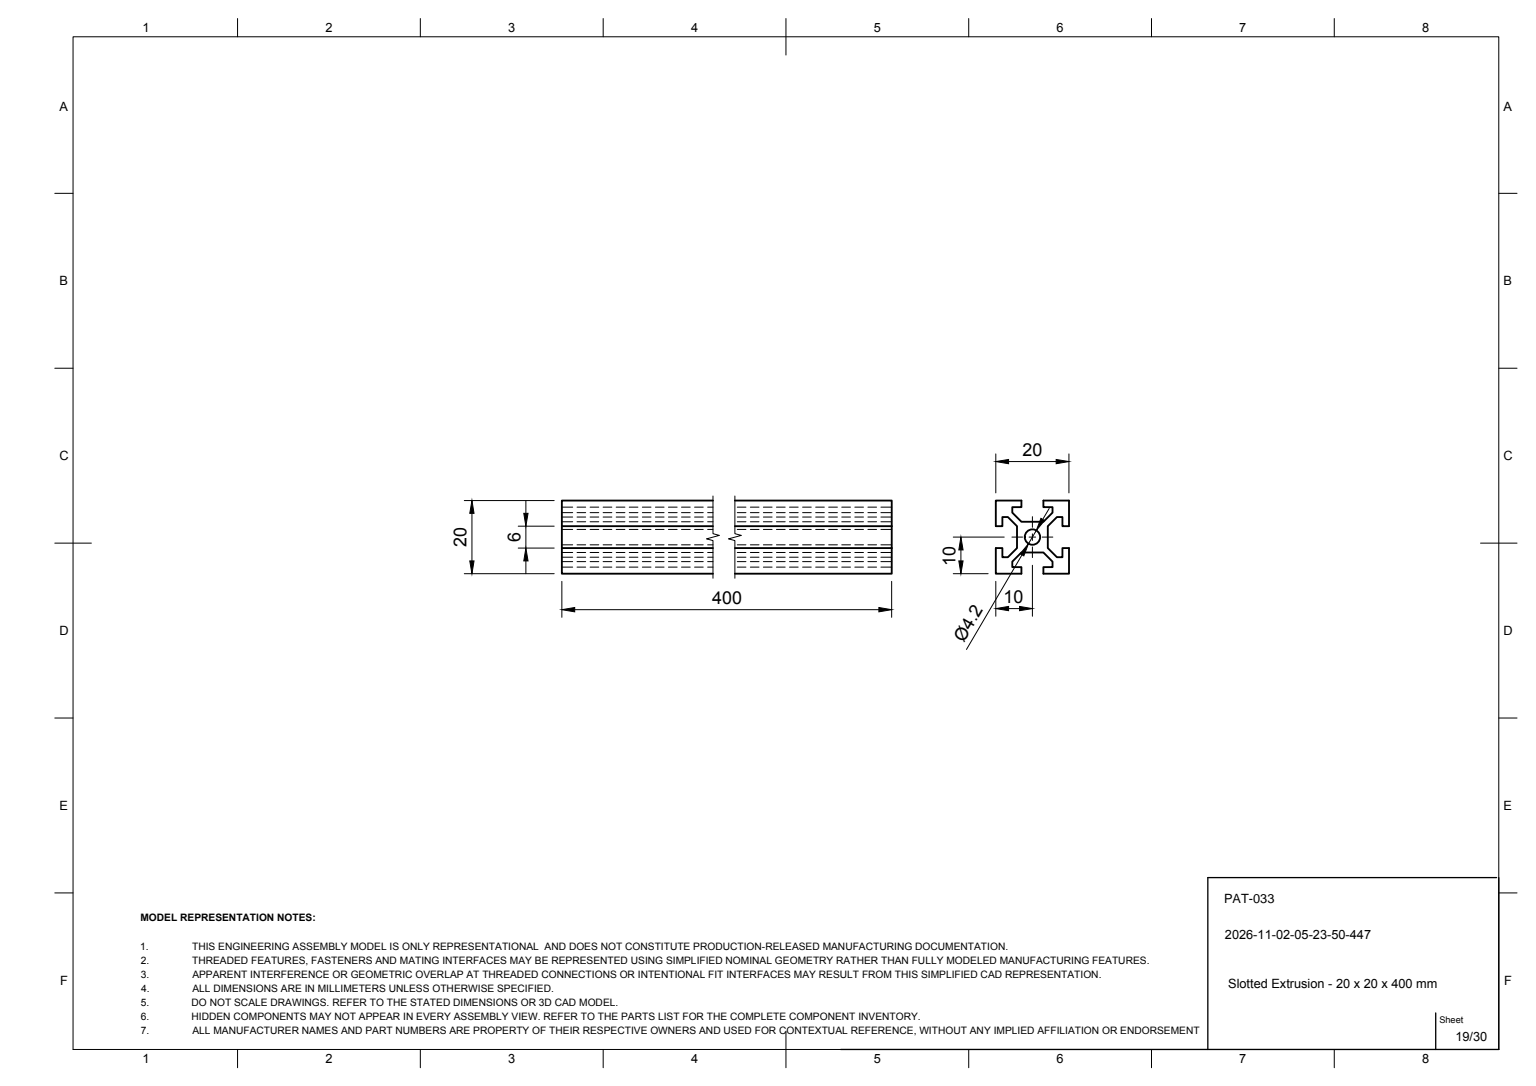
ISO-10303-21;
HEADER;
/* Generated by software containing ST-Developer
 * from STEP Tools, Inc. (www.steptools.com) 
 */

FILE_DESCRIPTION(
/* description */ ('Dual-rail gantry carriage'),
/* implementation_level */ '2;1');

FILE_NAME(
/* name */ 'Slotted Extrusion - 20 x 20 x 400 mm.step',
/* time_stamp */ '2026-10-27T10:49:15-07:00',
/* author */ (''),
/* organization */ (''),
/* preprocessor_version */ 'ST-DEVELOPER v20.2',
/* originating_system */ 'Autodesk Translation Framework v15.17.0.0',
/* authorisation */ '');

FILE_SCHEMA (('AUTOMOTIVE_DESIGN { 1 0 10303 214 3 1 1 }'));
ENDSEC;

DATA;
#10=MECHANICAL_DESIGN_GEOMETRIC_PRESENTATION_REPRESENTATION('',(#599),#12804);
#537=SHAPE_REPRESENTATION_RELATIONSHIP('SRR','None',#13015,#568);
#568=ADVANCED_BREP_SHAPE_REPRESENTATION('',(#630),#12785);
#599=STYLED_ITEM('',(#13233),#630);
#630=MANIFOLD_SOLID_BREP('Body1',#7377);
#690=FACE_BOUND('',#1655,.T.);
#691=FACE_BOUND('',#1657,.T.);
#856=PLANE('',#7946);
#857=PLANE('',#7947);
#858=PLANE('',#7948);
#859=PLANE('',#7949);
#860=PLANE('',#7950);
#861=PLANE('',#7951);
#862=PLANE('',#7952);
#863=PLANE('',#7953);
#864=PLANE('',#7954);
#865=PLANE('',#7955);
#866=PLANE('',#7956);
#867=PLANE('',#7957);
#868=PLANE('',#7958);
#869=PLANE('',#7959);
#870=PLANE('',#7960);
#871=PLANE('',#7961);
#872=PLANE('',#7962);
#873=PLANE('',#7963);
#874=PLANE('',#7964);
#875=PLANE('',#7965);
#876=PLANE('',#7966);
#877=PLANE('',#7967);
#878=PLANE('',#7968);
#879=PLANE('',#7969);
#880=PLANE('',#7970);
#881=PLANE('',#7971);
#882=PLANE('',#7972);
#883=PLANE('',#7973);
#884=PLANE('',#7974);
#885=PLANE('',#7975);
#886=PLANE('',#7976);
#887=PLANE('',#7977);
#888=PLANE('',#7978);
#889=PLANE('',#7979);
#890=PLANE('',#7980);
#891=PLANE('',#7981);
#892=PLANE('',#7985);
#893=PLANE('',#7986);
#894=PLANE('',#7987);
#895=PLANE('',#7988);
#896=PLANE('',#7989);
#897=PLANE('',#7990);
#898=PLANE('',#7991);
#899=PLANE('',#7992);
#900=PLANE('',#7993);
#901=PLANE('',#7994);
#1172=FACE_OUTER_BOUND('',#1609,.T.);
#1173=FACE_OUTER_BOUND('',#1610,.T.);
#1174=FACE_OUTER_BOUND('',#1611,.T.);
#1175=FACE_OUTER_BOUND('',#1612,.T.);
#1176=FACE_OUTER_BOUND('',#1613,.T.);
#1177=FACE_OUTER_BOUND('',#1614,.T.);
#1178=FACE_OUTER_BOUND('',#1615,.T.);
#1179=FACE_OUTER_BOUND('',#1616,.T.);
#1180=FACE_OUTER_BOUND('',#1617,.T.);
#1181=FACE_OUTER_BOUND('',#1618,.T.);
#1182=FACE_OUTER_BOUND('',#1619,.T.);
#1183=FACE_OUTER_BOUND('',#1620,.T.);
#1184=FACE_OUTER_BOUND('',#1621,.T.);
#1185=FACE_OUTER_BOUND('',#1622,.T.);
#1186=FACE_OUTER_BOUND('',#1623,.T.);
#1187=FACE_OUTER_BOUND('',#1624,.T.);
#1188=FACE_OUTER_BOUND('',#1625,.T.);
#1189=FACE_OUTER_BOUND('',#1626,.T.);
#1190=FACE_OUTER_BOUND('',#1627,.T.);
#1191=FACE_OUTER_BOUND('',#1628,.T.);
#1192=FACE_OUTER_BOUND('',#1629,.T.);
#1193=FACE_OUTER_BOUND('',#1630,.T.);
#1194=FACE_OUTER_BOUND('',#1631,.T.);
#1195=FACE_OUTER_BOUND('',#1632,.T.);
#1196=FACE_OUTER_BOUND('',#1633,.T.);
#1197=FACE_OUTER_BOUND('',#1634,.T.);
#1198=FACE_OUTER_BOUND('',#1635,.T.);
#1199=FACE_OUTER_BOUND('',#1636,.T.);
#1200=FACE_OUTER_BOUND('',#1637,.T.);
#1201=FACE_OUTER_BOUND('',#1638,.T.);
#1202=FACE_OUTER_BOUND('',#1639,.T.);
#1203=FACE_OUTER_BOUND('',#1640,.T.);
#1204=FACE_OUTER_BOUND('',#1641,.T.);
#1205=FACE_OUTER_BOUND('',#1642,.T.);
#1206=FACE_OUTER_BOUND('',#1643,.T.);
#1207=FACE_OUTER_BOUND('',#1644,.T.);
#1208=FACE_OUTER_BOUND('',#1645,.T.);
#1209=FACE_OUTER_BOUND('',#1646,.T.);
#1210=FACE_OUTER_BOUND('',#1647,.T.);
#1211=FACE_OUTER_BOUND('',#1648,.T.);
#1212=FACE_OUTER_BOUND('',#1649,.T.);
#1213=FACE_OUTER_BOUND('',#1650,.T.);
#1214=FACE_OUTER_BOUND('',#1651,.T.);
#1215=FACE_OUTER_BOUND('',#1652,.T.);
#1216=FACE_OUTER_BOUND('',#1653,.T.);
#1217=FACE_OUTER_BOUND('',#1654,.T.);
#1218=FACE_OUTER_BOUND('',#1656,.T.);
#1609=EDGE_LOOP('',(#5627,#5628,#5629,#5630));
#1610=EDGE_LOOP('',(#5631,#5632,#5633,#5634));
#1611=EDGE_LOOP('',(#5635,#5636,#5637,#5638));
#1612=EDGE_LOOP('',(#5639,#5640,#5641,#5642));
#1613=EDGE_LOOP('',(#5643,#5644,#5645,#5646));
#1614=EDGE_LOOP('',(#5647,#5648,#5649,#5650));
#1615=EDGE_LOOP('',(#5651,#5652,#5653,#5654));
#1616=EDGE_LOOP('',(#5655,#5656,#5657,#5658));
#1617=EDGE_LOOP('',(#5659,#5660,#5661,#5662));
#1618=EDGE_LOOP('',(#5663,#5664,#5665,#5666));
#1619=EDGE_LOOP('',(#5667,#5668,#5669,#5670));
#1620=EDGE_LOOP('',(#5671,#5672,#5673,#5674));
#1621=EDGE_LOOP('',(#5675,#5676,#5677,#5678));
#1622=EDGE_LOOP('',(#5679,#5680,#5681,#5682));
#1623=EDGE_LOOP('',(#5683,#5684,#5685,#5686));
#1624=EDGE_LOOP('',(#5687,#5688,#5689,#5690));
#1625=EDGE_LOOP('',(#5691,#5692,#5693,#5694));
#1626=EDGE_LOOP('',(#5695,#5696,#5697,#5698));
#1627=EDGE_LOOP('',(#5699,#5700,#5701,#5702));
#1628=EDGE_LOOP('',(#5703,#5704,#5705,#5706));
#1629=EDGE_LOOP('',(#5707,#5708,#5709,#5710));
#1630=EDGE_LOOP('',(#5711,#5712,#5713,#5714));
#1631=EDGE_LOOP('',(#5715,#5716,#5717,#5718));
#1632=EDGE_LOOP('',(#5719,#5720,#5721,#5722));
#1633=EDGE_LOOP('',(#5723,#5724,#5725,#5726));
#1634=EDGE_LOOP('',(#5727,#5728,#5729,#5730));
#1635=EDGE_LOOP('',(#5731,#5732,#5733,#5734));
#1636=EDGE_LOOP('',(#5735,#5736,#5737,#5738));
#1637=EDGE_LOOP('',(#5739,#5740,#5741,#5742));
#1638=EDGE_LOOP('',(#5743,#5744,#5745,#5746));
#1639=EDGE_LOOP('',(#5747,#5748,#5749,#5750));
#1640=EDGE_LOOP('',(#5751,#5752,#5753,#5754));
#1641=EDGE_LOOP('',(#5755,#5756,#5757,#5758));
#1642=EDGE_LOOP('',(#5759,#5760,#5761,#5762));
#1643=EDGE_LOOP('',(#5763,#5764,#5765,#5766));
#1644=EDGE_LOOP('',(#5767,#5768,#5769,#5770));
#1645=EDGE_LOOP('',(#5771,#5772,#5773,#5774));
#1646=EDGE_LOOP('',(#5775,#5776,#5777,#5778));
#1647=EDGE_LOOP('',(#5779,#5780,#5781,#5782));
#1648=EDGE_LOOP('',(#5783,#5784,#5785,#5786));
#1649=EDGE_LOOP('',(#5787,#5788,#5789,#5790));
#1650=EDGE_LOOP('',(#5791,#5792,#5793,#5794));
#1651=EDGE_LOOP('',(#5795,#5796,#5797,#5798));
#1652=EDGE_LOOP('',(#5799,#5800,#5801,#5802));
#1653=EDGE_LOOP('',(#5803,#5804,#5805,#5806));
#1654=EDGE_LOOP('',(#5807,#5808,#5809,#5810,#5811,#5812,#5813,#5814,#5815,
#5816,#5817,#5818,#5819,#5820,#5821,#5822,#5823,#5824,#5825,#5826,#5827,
#5828,#5829,#5830,#5831,#5832,#5833,#5834,#5835,#5836,#5837,#5838,#5839,
#5840,#5841,#5842,#5843,#5844,#5845,#5846,#5847,#5848,#5849,#5850));
#1655=EDGE_LOOP('',(#5851));
#1656=EDGE_LOOP('',(#5852,#5853,#5854,#5855,#5856,#5857,#5858,#5859,#5860,
#5861,#5862,#5863,#5864,#5865,#5866,#5867,#5868,#5869,#5870,#5871,#5872,
#5873,#5874,#5875,#5876,#5877,#5878,#5879,#5880,#5881,#5882,#5883,#5884,
#5885,#5886,#5887,#5888,#5889,#5890,#5891,#5892,#5893,#5894,#5895));
#1657=EDGE_LOOP('',(#5896));
#2164=LINE('',#11288,#2873);
#2165=LINE('',#11290,#2874);
#2166=LINE('',#11292,#2875);
#2167=LINE('',#11293,#2876);
#2168=LINE('',#11296,#2877);
#2169=LINE('',#11298,#2878);
#2170=LINE('',#11299,#2879);
#2171=LINE('',#11302,#2880);
#2172=LINE('',#11304,#2881);
#2173=LINE('',#11305,#2882);
#2174=LINE('',#11308,#2883);
#2175=LINE('',#11310,#2884);
#2176=LINE('',#11311,#2885);
#2177=LINE('',#11314,#2886);
#2178=LINE('',#11316,#2887);
#2179=LINE('',#11317,#2888);
#2180=LINE('',#11320,#2889);
#2181=LINE('',#11322,#2890);
#2182=LINE('',#11323,#2891);
#2183=LINE('',#11326,#2892);
#2184=LINE('',#11328,#2893);
#2185=LINE('',#11329,#2894);
#2186=LINE('',#11332,#2895);
#2187=LINE('',#11334,#2896);
#2188=LINE('',#11335,#2897);
#2189=LINE('',#11338,#2898);
#2190=LINE('',#11340,#2899);
#2191=LINE('',#11341,#2900);
#2192=LINE('',#11345,#2901);
#2193=LINE('',#11347,#2902);
#2194=LINE('',#11349,#2903);
#2195=LINE('',#11350,#2904);
#2196=LINE('',#11353,#2905);
#2197=LINE('',#11355,#2906);
#2198=LINE('',#11356,#2907);
#2199=LINE('',#11359,#2908);
#2200=LINE('',#11361,#2909);
#2201=LINE('',#11362,#2910);
#2202=LINE('',#11365,#2911);
#2203=LINE('',#11367,#2912);
#2204=LINE('',#11368,#2913);
#2205=LINE('',#11371,#2914);
#2206=LINE('',#11373,#2915);
#2207=LINE('',#11374,#2916);
#2208=LINE('',#11377,#2917);
#2209=LINE('',#11379,#2918);
#2210=LINE('',#11380,#2919);
#2211=LINE('',#11383,#2920);
#2212=LINE('',#11385,#2921);
#2213=LINE('',#11386,#2922);
#2214=LINE('',#11389,#2923);
#2215=LINE('',#11391,#2924);
#2216=LINE('',#11392,#2925);
#2217=LINE('',#11395,#2926);
#2218=LINE('',#11397,#2927);
#2219=LINE('',#11398,#2928);
#2220=LINE('',#11402,#2929);
#2221=LINE('',#11404,#2930);
#2222=LINE('',#11406,#2931);
#2223=LINE('',#11407,#2932);
#2224=LINE('',#11410,#2933);
#2225=LINE('',#11412,#2934);
#2226=LINE('',#11413,#2935);
#2227=LINE('',#11416,#2936);
#2228=LINE('',#11418,#2937);
#2229=LINE('',#11419,#2938);
#2230=LINE('',#11422,#2939);
#2231=LINE('',#11424,#2940);
#2232=LINE('',#11425,#2941);
#2233=LINE('',#11428,#2942);
#2234=LINE('',#11430,#2943);
#2235=LINE('',#11431,#2944);
#2236=LINE('',#11434,#2945);
#2237=LINE('',#11436,#2946);
#2238=LINE('',#11437,#2947);
#2239=LINE('',#11440,#2948);
#2240=LINE('',#11442,#2949);
#2241=LINE('',#11443,#2950);
#2242=LINE('',#11446,#2951);
#2243=LINE('',#11448,#2952);
#2244=LINE('',#11449,#2953);
#2245=LINE('',#11452,#2954);
#2246=LINE('',#11454,#2955);
#2247=LINE('',#11455,#2956);
#2248=LINE('',#11459,#2957);
#2249=LINE('',#11461,#2958);
#2250=LINE('',#11463,#2959);
#2251=LINE('',#11464,#2960);
#2252=LINE('',#11467,#2961);
#2253=LINE('',#11469,#2962);
#2254=LINE('',#11470,#2963);
#2255=LINE('',#11473,#2964);
#2256=LINE('',#11475,#2965);
#2257=LINE('',#11476,#2966);
#2258=LINE('',#11479,#2967);
#2259=LINE('',#11481,#2968);
#2260=LINE('',#11482,#2969);
#2261=LINE('',#11485,#2970);
#2262=LINE('',#11487,#2971);
#2263=LINE('',#11488,#2972);
#2264=LINE('',#11491,#2973);
#2265=LINE('',#11493,#2974);
#2266=LINE('',#11494,#2975);
#2267=LINE('',#11497,#2976);
#2268=LINE('',#11499,#2977);
#2269=LINE('',#11500,#2978);
#2270=LINE('',#11503,#2979);
#2271=LINE('',#11505,#2980);
#2272=LINE('',#11506,#2981);
#2273=LINE('',#11509,#2982);
#2274=LINE('',#11511,#2983);
#2275=LINE('',#11512,#2984);
#2276=LINE('',#11517,#2985);
#2277=LINE('',#11521,#2986);
#2278=LINE('',#11523,#2987);
#2279=LINE('',#11524,#2988);
#2280=LINE('',#11527,#2989);
#2281=LINE('',#11529,#2990);
#2282=LINE('',#11530,#2991);
#2283=LINE('',#11532,#2992);
#2284=LINE('',#11533,#2993);
#2285=LINE('',#11536,#2994);
#2286=LINE('',#11538,#2995);
#2287=LINE('',#11539,#2996);
#2288=LINE('',#11541,#2997);
#2289=LINE('',#11542,#2998);
#2290=LINE('',#11545,#2999);
#2291=LINE('',#11547,#3000);
#2292=LINE('',#11548,#3001);
#2293=LINE('',#11550,#3002);
#2294=LINE('',#11551,#3003);
#2295=LINE('',#11553,#3004);
#2296=LINE('',#11554,#3005);
#2873=VECTOR('',#9115,1.);
#2874=VECTOR('',#9116,1.);
#2875=VECTOR('',#9117,1.);
#2876=VECTOR('',#9118,1.);
#2877=VECTOR('',#9121,1.);
#2878=VECTOR('',#9122,1.);
#2879=VECTOR('',#9123,1.);
#2880=VECTOR('',#9126,1.);
#2881=VECTOR('',#9127,1.);
#2882=VECTOR('',#9128,1.);
#2883=VECTOR('',#9131,1.);
#2884=VECTOR('',#9132,1.);
#2885=VECTOR('',#9133,1.);
#2886=VECTOR('',#9136,1.);
#2887=VECTOR('',#9137,1.);
#2888=VECTOR('',#9138,1.);
#2889=VECTOR('',#9141,1.);
#2890=VECTOR('',#9142,1.);
#2891=VECTOR('',#9143,1.);
#2892=VECTOR('',#9146,1.);
#2893=VECTOR('',#9147,1.);
#2894=VECTOR('',#9148,1.);
#2895=VECTOR('',#9151,1.);
#2896=VECTOR('',#9152,1.);
#2897=VECTOR('',#9153,1.);
#2898=VECTOR('',#9156,1.);
#2899=VECTOR('',#9157,1.);
#2900=VECTOR('',#9158,1.);
#2901=VECTOR('',#9161,1.);
#2902=VECTOR('',#9162,1.);
#2903=VECTOR('',#9163,1.);
#2904=VECTOR('',#9164,1.);
#2905=VECTOR('',#9167,1.);
#2906=VECTOR('',#9168,1.);
#2907=VECTOR('',#9169,1.);
#2908=VECTOR('',#9172,1.);
#2909=VECTOR('',#9173,1.);
#2910=VECTOR('',#9174,1.);
#2911=VECTOR('',#9177,1.);
#2912=VECTOR('',#9178,1.);
#2913=VECTOR('',#9179,1.);
#2914=VECTOR('',#9182,1.);
#2915=VECTOR('',#9183,1.);
#2916=VECTOR('',#9184,1.);
#2917=VECTOR('',#9187,1.);
#2918=VECTOR('',#9188,1.);
#2919=VECTOR('',#9189,1.);
#2920=VECTOR('',#9192,1.);
#2921=VECTOR('',#9193,1.);
#2922=VECTOR('',#9194,1.);
#2923=VECTOR('',#9197,1.);
#2924=VECTOR('',#9198,1.);
#2925=VECTOR('',#9199,1.);
#2926=VECTOR('',#9202,1.);
#2927=VECTOR('',#9203,1.);
#2928=VECTOR('',#9204,1.);
#2929=VECTOR('',#9207,1.);
#2930=VECTOR('',#9208,1.);
#2931=VECTOR('',#9209,1.);
#2932=VECTOR('',#9210,1.);
#2933=VECTOR('',#9213,1.);
#2934=VECTOR('',#9214,1.);
#2935=VECTOR('',#9215,1.);
#2936=VECTOR('',#9218,1.);
#2937=VECTOR('',#9219,1.);
#2938=VECTOR('',#9220,1.);
#2939=VECTOR('',#9223,1.);
#2940=VECTOR('',#9224,1.);
#2941=VECTOR('',#9225,1.);
#2942=VECTOR('',#9228,1.);
#2943=VECTOR('',#9229,1.);
#2944=VECTOR('',#9230,1.);
#2945=VECTOR('',#9233,1.);
#2946=VECTOR('',#9234,1.);
#2947=VECTOR('',#9235,1.);
#2948=VECTOR('',#9238,1.);
#2949=VECTOR('',#9239,1.);
#2950=VECTOR('',#9240,1.);
#2951=VECTOR('',#9243,1.);
#2952=VECTOR('',#9244,1.);
#2953=VECTOR('',#9245,1.);
#2954=VECTOR('',#9248,1.);
#2955=VECTOR('',#9249,1.);
#2956=VECTOR('',#9250,1.);
#2957=VECTOR('',#9253,1.);
#2958=VECTOR('',#9254,1.);
#2959=VECTOR('',#9255,1.);
#2960=VECTOR('',#9256,1.);
#2961=VECTOR('',#9259,1.);
#2962=VECTOR('',#9260,1.);
#2963=VECTOR('',#9261,1.);
#2964=VECTOR('',#9264,1.);
#2965=VECTOR('',#9265,1.);
#2966=VECTOR('',#9266,1.);
#2967=VECTOR('',#9269,1.);
#2968=VECTOR('',#9270,1.);
#2969=VECTOR('',#9271,1.);
#2970=VECTOR('',#9274,1.);
#2971=VECTOR('',#9275,1.);
#2972=VECTOR('',#9276,1.);
#2973=VECTOR('',#9279,1.);
#2974=VECTOR('',#9280,1.);
#2975=VECTOR('',#9281,1.);
#2976=VECTOR('',#9284,1.);
#2977=VECTOR('',#9285,1.);
#2978=VECTOR('',#9286,1.);
#2979=VECTOR('',#9289,1.);
#2980=VECTOR('',#9290,1.);
#2981=VECTOR('',#9291,1.);
#2982=VECTOR('',#9294,1.);
#2983=VECTOR('',#9295,1.);
#2984=VECTOR('',#9296,1.);
#2985=VECTOR('',#9301,0.21);
#2986=VECTOR('',#9306,1.);
#2987=VECTOR('',#9307,1.);
#2988=VECTOR('',#9308,1.);
#2989=VECTOR('',#9311,1.);
#2990=VECTOR('',#9312,1.);
#2991=VECTOR('',#9313,1.);
#2992=VECTOR('',#9316,1.);
#2993=VECTOR('',#9317,1.);
#2994=VECTOR('',#9320,1.);
#2995=VECTOR('',#9321,1.);
#2996=VECTOR('',#9322,1.);
#2997=VECTOR('',#9325,1.);
#2998=VECTOR('',#9326,1.);
#2999=VECTOR('',#9329,1.);
#3000=VECTOR('',#9330,1.);
#3001=VECTOR('',#9331,1.);
#3002=VECTOR('',#9334,1.);
#3003=VECTOR('',#9335,1.);
#3004=VECTOR('',#9338,1.);
#3005=VECTOR('',#9339,1.);
#3430=CIRCLE('',#7983,0.21);
#3431=CIRCLE('',#7984,0.21);
#3742=VERTEX_POINT('',#11286);
#3743=VERTEX_POINT('',#11287);
#3744=VERTEX_POINT('',#11289);
#3745=VERTEX_POINT('',#11291);
#3746=VERTEX_POINT('',#11295);
#3747=VERTEX_POINT('',#11297);
#3748=VERTEX_POINT('',#11301);
#3749=VERTEX_POINT('',#11303);
#3750=VERTEX_POINT('',#11307);
#3751=VERTEX_POINT('',#11309);
#3752=VERTEX_POINT('',#11313);
#3753=VERTEX_POINT('',#11315);
#3754=VERTEX_POINT('',#11319);
#3755=VERTEX_POINT('',#11321);
#3756=VERTEX_POINT('',#11325);
#3757=VERTEX_POINT('',#11327);
#3758=VERTEX_POINT('',#11331);
#3759=VERTEX_POINT('',#11333);
#3760=VERTEX_POINT('',#11337);
#3761=VERTEX_POINT('',#11339);
#3762=VERTEX_POINT('',#11343);
#3763=VERTEX_POINT('',#11344);
#3764=VERTEX_POINT('',#11346);
#3765=VERTEX_POINT('',#11348);
#3766=VERTEX_POINT('',#11352);
#3767=VERTEX_POINT('',#11354);
#3768=VERTEX_POINT('',#11358);
#3769=VERTEX_POINT('',#11360);
#3770=VERTEX_POINT('',#11364);
#3771=VERTEX_POINT('',#11366);
#3772=VERTEX_POINT('',#11370);
#3773=VERTEX_POINT('',#11372);
#3774=VERTEX_POINT('',#11376);
#3775=VERTEX_POINT('',#11378);
#3776=VERTEX_POINT('',#11382);
#3777=VERTEX_POINT('',#11384);
#3778=VERTEX_POINT('',#11388);
#3779=VERTEX_POINT('',#11390);
#3780=VERTEX_POINT('',#11394);
#3781=VERTEX_POINT('',#11396);
#3782=VERTEX_POINT('',#11400);
#3783=VERTEX_POINT('',#11401);
#3784=VERTEX_POINT('',#11403);
#3785=VERTEX_POINT('',#11405);
#3786=VERTEX_POINT('',#11409);
#3787=VERTEX_POINT('',#11411);
#3788=VERTEX_POINT('',#11415);
#3789=VERTEX_POINT('',#11417);
#3790=VERTEX_POINT('',#11421);
#3791=VERTEX_POINT('',#11423);
#3792=VERTEX_POINT('',#11427);
#3793=VERTEX_POINT('',#11429);
#3794=VERTEX_POINT('',#11433);
#3795=VERTEX_POINT('',#11435);
#3796=VERTEX_POINT('',#11439);
#3797=VERTEX_POINT('',#11441);
#3798=VERTEX_POINT('',#11445);
#3799=VERTEX_POINT('',#11447);
#3800=VERTEX_POINT('',#11451);
#3801=VERTEX_POINT('',#11453);
#3802=VERTEX_POINT('',#11457);
#3803=VERTEX_POINT('',#11458);
#3804=VERTEX_POINT('',#11460);
#3805=VERTEX_POINT('',#11462);
#3806=VERTEX_POINT('',#11466);
#3807=VERTEX_POINT('',#11468);
#3808=VERTEX_POINT('',#11472);
#3809=VERTEX_POINT('',#11474);
#3810=VERTEX_POINT('',#11478);
#3811=VERTEX_POINT('',#11480);
#3812=VERTEX_POINT('',#11484);
#3813=VERTEX_POINT('',#11486);
#3814=VERTEX_POINT('',#11490);
#3815=VERTEX_POINT('',#11492);
#3816=VERTEX_POINT('',#11496);
#3817=VERTEX_POINT('',#11498);
#3818=VERTEX_POINT('',#11502);
#3819=VERTEX_POINT('',#11504);
#3820=VERTEX_POINT('',#11508);
#3821=VERTEX_POINT('',#11510);
#3822=VERTEX_POINT('',#11514);
#3823=VERTEX_POINT('',#11516);
#3824=VERTEX_POINT('',#11520);
#3825=VERTEX_POINT('',#11522);
#3826=VERTEX_POINT('',#11526);
#3827=VERTEX_POINT('',#11528);
#3828=VERTEX_POINT('',#11535);
#3829=VERTEX_POINT('',#11537);
#3830=VERTEX_POINT('',#11544);
#3831=VERTEX_POINT('',#11546);
#4436=EDGE_CURVE('',#3742,#3743,#2164,.T.);
#4437=EDGE_CURVE('',#3742,#3744,#2165,.T.);
#4438=EDGE_CURVE('',#3745,#3744,#2166,.T.);
#4439=EDGE_CURVE('',#3743,#3745,#2167,.T.);
#4440=EDGE_CURVE('',#3746,#3742,#2168,.T.);
#4441=EDGE_CURVE('',#3746,#3747,#2169,.T.);
#4442=EDGE_CURVE('',#3744,#3747,#2170,.T.);
#4443=EDGE_CURVE('',#3748,#3746,#2171,.T.);
#4444=EDGE_CURVE('',#3748,#3749,#2172,.T.);
#4445=EDGE_CURVE('',#3747,#3749,#2173,.T.);
#4446=EDGE_CURVE('',#3750,#3748,#2174,.T.);
#4447=EDGE_CURVE('',#3750,#3751,#2175,.T.);
#4448=EDGE_CURVE('',#3749,#3751,#2176,.T.);
#4449=EDGE_CURVE('',#3752,#3750,#2177,.T.);
#4450=EDGE_CURVE('',#3752,#3753,#2178,.T.);
#4451=EDGE_CURVE('',#3751,#3753,#2179,.T.);
#4452=EDGE_CURVE('',#3754,#3752,#2180,.T.);
#4453=EDGE_CURVE('',#3754,#3755,#2181,.T.);
#4454=EDGE_CURVE('',#3753,#3755,#2182,.T.);
#4455=EDGE_CURVE('',#3756,#3754,#2183,.T.);
#4456=EDGE_CURVE('',#3756,#3757,#2184,.T.);
#4457=EDGE_CURVE('',#3755,#3757,#2185,.T.);
#4458=EDGE_CURVE('',#3758,#3756,#2186,.T.);
#4459=EDGE_CURVE('',#3758,#3759,#2187,.T.);
#4460=EDGE_CURVE('',#3757,#3759,#2188,.T.);
#4461=EDGE_CURVE('',#3760,#3758,#2189,.T.);
#4462=EDGE_CURVE('',#3761,#3760,#2190,.T.);
#4463=EDGE_CURVE('',#3759,#3761,#2191,.T.);
#4464=EDGE_CURVE('',#3762,#3763,#2192,.T.);
#4465=EDGE_CURVE('',#3762,#3764,#2193,.T.);
#4466=EDGE_CURVE('',#3765,#3764,#2194,.T.);
#4467=EDGE_CURVE('',#3763,#3765,#2195,.T.);
#4468=EDGE_CURVE('',#3766,#3762,#2196,.T.);
#4469=EDGE_CURVE('',#3766,#3767,#2197,.T.);
#4470=EDGE_CURVE('',#3764,#3767,#2198,.T.);
#4471=EDGE_CURVE('',#3768,#3766,#2199,.T.);
#4472=EDGE_CURVE('',#3768,#3769,#2200,.T.);
#4473=EDGE_CURVE('',#3767,#3769,#2201,.T.);
#4474=EDGE_CURVE('',#3770,#3768,#2202,.T.);
#4475=EDGE_CURVE('',#3770,#3771,#2203,.T.);
#4476=EDGE_CURVE('',#3769,#3771,#2204,.T.);
#4477=EDGE_CURVE('',#3772,#3770,#2205,.T.);
#4478=EDGE_CURVE('',#3772,#3773,#2206,.T.);
#4479=EDGE_CURVE('',#3771,#3773,#2207,.T.);
#4480=EDGE_CURVE('',#3774,#3772,#2208,.T.);
#4481=EDGE_CURVE('',#3774,#3775,#2209,.T.);
#4482=EDGE_CURVE('',#3773,#3775,#2210,.T.);
#4483=EDGE_CURVE('',#3776,#3774,#2211,.T.);
#4484=EDGE_CURVE('',#3776,#3777,#2212,.T.);
#4485=EDGE_CURVE('',#3775,#3777,#2213,.T.);
#4486=EDGE_CURVE('',#3778,#3776,#2214,.T.);
#4487=EDGE_CURVE('',#3778,#3779,#2215,.T.);
#4488=EDGE_CURVE('',#3777,#3779,#2216,.T.);
#4489=EDGE_CURVE('',#3780,#3778,#2217,.T.);
#4490=EDGE_CURVE('',#3781,#3780,#2218,.T.);
#4491=EDGE_CURVE('',#3779,#3781,#2219,.T.);
#4492=EDGE_CURVE('',#3782,#3783,#2220,.T.);
#4493=EDGE_CURVE('',#3782,#3784,#2221,.T.);
#4494=EDGE_CURVE('',#3785,#3784,#2222,.T.);
#4495=EDGE_CURVE('',#3783,#3785,#2223,.T.);
#4496=EDGE_CURVE('',#3786,#3782,#2224,.T.);
#4497=EDGE_CURVE('',#3786,#3787,#2225,.T.);
#4498=EDGE_CURVE('',#3784,#3787,#2226,.T.);
#4499=EDGE_CURVE('',#3788,#3786,#2227,.T.);
#4500=EDGE_CURVE('',#3788,#3789,#2228,.T.);
#4501=EDGE_CURVE('',#3787,#3789,#2229,.T.);
#4502=EDGE_CURVE('',#3790,#3788,#2230,.T.);
#4503=EDGE_CURVE('',#3790,#3791,#2231,.T.);
#4504=EDGE_CURVE('',#3789,#3791,#2232,.T.);
#4505=EDGE_CURVE('',#3792,#3790,#2233,.T.);
#4506=EDGE_CURVE('',#3792,#3793,#2234,.T.);
#4507=EDGE_CURVE('',#3791,#3793,#2235,.T.);
#4508=EDGE_CURVE('',#3794,#3792,#2236,.T.);
#4509=EDGE_CURVE('',#3794,#3795,#2237,.T.);
#4510=EDGE_CURVE('',#3793,#3795,#2238,.T.);
#4511=EDGE_CURVE('',#3796,#3794,#2239,.T.);
#4512=EDGE_CURVE('',#3796,#3797,#2240,.T.);
#4513=EDGE_CURVE('',#3795,#3797,#2241,.T.);
#4514=EDGE_CURVE('',#3798,#3796,#2242,.T.);
#4515=EDGE_CURVE('',#3798,#3799,#2243,.T.);
#4516=EDGE_CURVE('',#3797,#3799,#2244,.T.);
#4517=EDGE_CURVE('',#3800,#3798,#2245,.T.);
#4518=EDGE_CURVE('',#3801,#3800,#2246,.T.);
#4519=EDGE_CURVE('',#3799,#3801,#2247,.T.);
#4520=EDGE_CURVE('',#3802,#3803,#2248,.T.);
#4521=EDGE_CURVE('',#3802,#3804,#2249,.T.);
#4522=EDGE_CURVE('',#3805,#3804,#2250,.T.);
#4523=EDGE_CURVE('',#3803,#3805,#2251,.T.);
#4524=EDGE_CURVE('',#3806,#3802,#2252,.T.);
#4525=EDGE_CURVE('',#3806,#3807,#2253,.T.);
#4526=EDGE_CURVE('',#3804,#3807,#2254,.T.);
#4527=EDGE_CURVE('',#3808,#3806,#2255,.T.);
#4528=EDGE_CURVE('',#3808,#3809,#2256,.T.);
#4529=EDGE_CURVE('',#3807,#3809,#2257,.T.);
#4530=EDGE_CURVE('',#3810,#3808,#2258,.T.);
#4531=EDGE_CURVE('',#3810,#3811,#2259,.T.);
#4532=EDGE_CURVE('',#3809,#3811,#2260,.T.);
#4533=EDGE_CURVE('',#3812,#3810,#2261,.T.);
#4534=EDGE_CURVE('',#3812,#3813,#2262,.T.);
#4535=EDGE_CURVE('',#3811,#3813,#2263,.T.);
#4536=EDGE_CURVE('',#3814,#3812,#2264,.T.);
#4537=EDGE_CURVE('',#3814,#3815,#2265,.T.);
#4538=EDGE_CURVE('',#3813,#3815,#2266,.T.);
#4539=EDGE_CURVE('',#3816,#3814,#2267,.T.);
#4540=EDGE_CURVE('',#3816,#3817,#2268,.T.);
#4541=EDGE_CURVE('',#3815,#3817,#2269,.T.);
#4542=EDGE_CURVE('',#3818,#3816,#2270,.T.);
#4543=EDGE_CURVE('',#3818,#3819,#2271,.T.);
#4544=EDGE_CURVE('',#3817,#3819,#2272,.T.);
#4545=EDGE_CURVE('',#3820,#3818,#2273,.T.);
#4546=EDGE_CURVE('',#3821,#3820,#2274,.T.);
#4547=EDGE_CURVE('',#3819,#3821,#2275,.T.);
#4548=EDGE_CURVE('',#3822,#3822,#3430,.T.);
#4549=EDGE_CURVE('',#3822,#3823,#2276,.T.);
#4550=EDGE_CURVE('',#3823,#3823,#3431,.T.);
#4551=EDGE_CURVE('',#3760,#3824,#2277,.T.);
#4552=EDGE_CURVE('',#3824,#3825,#2278,.T.);
#4553=EDGE_CURVE('',#3761,#3825,#2279,.T.);
#4554=EDGE_CURVE('',#3826,#3745,#2280,.T.);
#4555=EDGE_CURVE('',#3827,#3826,#2281,.T.);
#4556=EDGE_CURVE('',#3827,#3743,#2282,.T.);
#4557=EDGE_CURVE('',#3780,#3827,#2283,.T.);
#4558=EDGE_CURVE('',#3781,#3826,#2284,.T.);
#4559=EDGE_CURVE('',#3828,#3765,#2285,.T.);
#4560=EDGE_CURVE('',#3829,#3828,#2286,.T.);
#4561=EDGE_CURVE('',#3829,#3763,#2287,.T.);
#4562=EDGE_CURVE('',#3800,#3829,#2288,.T.);
#4563=EDGE_CURVE('',#3801,#3828,#2289,.T.);
#4564=EDGE_CURVE('',#3830,#3785,#2290,.T.);
#4565=EDGE_CURVE('',#3831,#3830,#2291,.T.);
#4566=EDGE_CURVE('',#3831,#3783,#2292,.T.);
#4567=EDGE_CURVE('',#3820,#3831,#2293,.T.);
#4568=EDGE_CURVE('',#3821,#3830,#2294,.T.);
#4569=EDGE_CURVE('',#3825,#3805,#2295,.T.);
#4570=EDGE_CURVE('',#3824,#3803,#2296,.T.);
#5627=ORIENTED_EDGE('',*,*,#4436,.F.);
#5628=ORIENTED_EDGE('',*,*,#4437,.T.);
#5629=ORIENTED_EDGE('',*,*,#4438,.F.);
#5630=ORIENTED_EDGE('',*,*,#4439,.F.);
#5631=ORIENTED_EDGE('',*,*,#4440,.F.);
#5632=ORIENTED_EDGE('',*,*,#4441,.T.);
#5633=ORIENTED_EDGE('',*,*,#4442,.F.);
#5634=ORIENTED_EDGE('',*,*,#4437,.F.);
#5635=ORIENTED_EDGE('',*,*,#4443,.F.);
#5636=ORIENTED_EDGE('',*,*,#4444,.T.);
#5637=ORIENTED_EDGE('',*,*,#4445,.F.);
#5638=ORIENTED_EDGE('',*,*,#4441,.F.);
#5639=ORIENTED_EDGE('',*,*,#4446,.F.);
#5640=ORIENTED_EDGE('',*,*,#4447,.T.);
#5641=ORIENTED_EDGE('',*,*,#4448,.F.);
#5642=ORIENTED_EDGE('',*,*,#4444,.F.);
#5643=ORIENTED_EDGE('',*,*,#4449,.F.);
#5644=ORIENTED_EDGE('',*,*,#4450,.T.);
#5645=ORIENTED_EDGE('',*,*,#4451,.F.);
#5646=ORIENTED_EDGE('',*,*,#4447,.F.);
#5647=ORIENTED_EDGE('',*,*,#4452,.F.);
#5648=ORIENTED_EDGE('',*,*,#4453,.T.);
#5649=ORIENTED_EDGE('',*,*,#4454,.F.);
#5650=ORIENTED_EDGE('',*,*,#4450,.F.);
#5651=ORIENTED_EDGE('',*,*,#4455,.F.);
#5652=ORIENTED_EDGE('',*,*,#4456,.T.);
#5653=ORIENTED_EDGE('',*,*,#4457,.F.);
#5654=ORIENTED_EDGE('',*,*,#4453,.F.);
#5655=ORIENTED_EDGE('',*,*,#4458,.F.);
#5656=ORIENTED_EDGE('',*,*,#4459,.T.);
#5657=ORIENTED_EDGE('',*,*,#4460,.F.);
#5658=ORIENTED_EDGE('',*,*,#4456,.F.);
#5659=ORIENTED_EDGE('',*,*,#4461,.F.);
#5660=ORIENTED_EDGE('',*,*,#4462,.F.);
#5661=ORIENTED_EDGE('',*,*,#4463,.F.);
#5662=ORIENTED_EDGE('',*,*,#4459,.F.);
#5663=ORIENTED_EDGE('',*,*,#4464,.F.);
#5664=ORIENTED_EDGE('',*,*,#4465,.T.);
#5665=ORIENTED_EDGE('',*,*,#4466,.F.);
#5666=ORIENTED_EDGE('',*,*,#4467,.F.);
#5667=ORIENTED_EDGE('',*,*,#4468,.F.);
#5668=ORIENTED_EDGE('',*,*,#4469,.T.);
#5669=ORIENTED_EDGE('',*,*,#4470,.F.);
#5670=ORIENTED_EDGE('',*,*,#4465,.F.);
#5671=ORIENTED_EDGE('',*,*,#4471,.F.);
#5672=ORIENTED_EDGE('',*,*,#4472,.T.);
#5673=ORIENTED_EDGE('',*,*,#4473,.F.);
#5674=ORIENTED_EDGE('',*,*,#4469,.F.);
#5675=ORIENTED_EDGE('',*,*,#4474,.F.);
#5676=ORIENTED_EDGE('',*,*,#4475,.T.);
#5677=ORIENTED_EDGE('',*,*,#4476,.F.);
#5678=ORIENTED_EDGE('',*,*,#4472,.F.);
#5679=ORIENTED_EDGE('',*,*,#4477,.F.);
#5680=ORIENTED_EDGE('',*,*,#4478,.T.);
#5681=ORIENTED_EDGE('',*,*,#4479,.F.);
#5682=ORIENTED_EDGE('',*,*,#4475,.F.);
#5683=ORIENTED_EDGE('',*,*,#4480,.F.);
#5684=ORIENTED_EDGE('',*,*,#4481,.T.);
#5685=ORIENTED_EDGE('',*,*,#4482,.F.);
#5686=ORIENTED_EDGE('',*,*,#4478,.F.);
#5687=ORIENTED_EDGE('',*,*,#4483,.F.);
#5688=ORIENTED_EDGE('',*,*,#4484,.T.);
#5689=ORIENTED_EDGE('',*,*,#4485,.F.);
#5690=ORIENTED_EDGE('',*,*,#4481,.F.);
#5691=ORIENTED_EDGE('',*,*,#4486,.F.);
#5692=ORIENTED_EDGE('',*,*,#4487,.T.);
#5693=ORIENTED_EDGE('',*,*,#4488,.F.);
#5694=ORIENTED_EDGE('',*,*,#4484,.F.);
#5695=ORIENTED_EDGE('',*,*,#4489,.F.);
#5696=ORIENTED_EDGE('',*,*,#4490,.F.);
#5697=ORIENTED_EDGE('',*,*,#4491,.F.);
#5698=ORIENTED_EDGE('',*,*,#4487,.F.);
#5699=ORIENTED_EDGE('',*,*,#4492,.F.);
#5700=ORIENTED_EDGE('',*,*,#4493,.T.);
#5701=ORIENTED_EDGE('',*,*,#4494,.F.);
#5702=ORIENTED_EDGE('',*,*,#4495,.F.);
#5703=ORIENTED_EDGE('',*,*,#4496,.F.);
#5704=ORIENTED_EDGE('',*,*,#4497,.T.);
#5705=ORIENTED_EDGE('',*,*,#4498,.F.);
#5706=ORIENTED_EDGE('',*,*,#4493,.F.);
#5707=ORIENTED_EDGE('',*,*,#4499,.F.);
#5708=ORIENTED_EDGE('',*,*,#4500,.T.);
#5709=ORIENTED_EDGE('',*,*,#4501,.F.);
#5710=ORIENTED_EDGE('',*,*,#4497,.F.);
#5711=ORIENTED_EDGE('',*,*,#4502,.F.);
#5712=ORIENTED_EDGE('',*,*,#4503,.T.);
#5713=ORIENTED_EDGE('',*,*,#4504,.F.);
#5714=ORIENTED_EDGE('',*,*,#4500,.F.);
#5715=ORIENTED_EDGE('',*,*,#4505,.F.);
#5716=ORIENTED_EDGE('',*,*,#4506,.T.);
#5717=ORIENTED_EDGE('',*,*,#4507,.F.);
#5718=ORIENTED_EDGE('',*,*,#4503,.F.);
#5719=ORIENTED_EDGE('',*,*,#4508,.F.);
#5720=ORIENTED_EDGE('',*,*,#4509,.T.);
#5721=ORIENTED_EDGE('',*,*,#4510,.F.);
#5722=ORIENTED_EDGE('',*,*,#4506,.F.);
#5723=ORIENTED_EDGE('',*,*,#4511,.F.);
#5724=ORIENTED_EDGE('',*,*,#4512,.T.);
#5725=ORIENTED_EDGE('',*,*,#4513,.F.);
#5726=ORIENTED_EDGE('',*,*,#4509,.F.);
#5727=ORIENTED_EDGE('',*,*,#4514,.F.);
#5728=ORIENTED_EDGE('',*,*,#4515,.T.);
#5729=ORIENTED_EDGE('',*,*,#4516,.F.);
#5730=ORIENTED_EDGE('',*,*,#4512,.F.);
#5731=ORIENTED_EDGE('',*,*,#4517,.F.);
#5732=ORIENTED_EDGE('',*,*,#4518,.F.);
#5733=ORIENTED_EDGE('',*,*,#4519,.F.);
#5734=ORIENTED_EDGE('',*,*,#4515,.F.);
#5735=ORIENTED_EDGE('',*,*,#4520,.F.);
#5736=ORIENTED_EDGE('',*,*,#4521,.T.);
#5737=ORIENTED_EDGE('',*,*,#4522,.F.);
#5738=ORIENTED_EDGE('',*,*,#4523,.F.);
#5739=ORIENTED_EDGE('',*,*,#4524,.F.);
#5740=ORIENTED_EDGE('',*,*,#4525,.T.);
#5741=ORIENTED_EDGE('',*,*,#4526,.F.);
#5742=ORIENTED_EDGE('',*,*,#4521,.F.);
#5743=ORIENTED_EDGE('',*,*,#4527,.F.);
#5744=ORIENTED_EDGE('',*,*,#4528,.T.);
#5745=ORIENTED_EDGE('',*,*,#4529,.F.);
#5746=ORIENTED_EDGE('',*,*,#4525,.F.);
#5747=ORIENTED_EDGE('',*,*,#4530,.F.);
#5748=ORIENTED_EDGE('',*,*,#4531,.T.);
#5749=ORIENTED_EDGE('',*,*,#4532,.F.);
#5750=ORIENTED_EDGE('',*,*,#4528,.F.);
#5751=ORIENTED_EDGE('',*,*,#4533,.F.);
#5752=ORIENTED_EDGE('',*,*,#4534,.T.);
#5753=ORIENTED_EDGE('',*,*,#4535,.F.);
#5754=ORIENTED_EDGE('',*,*,#4531,.F.);
#5755=ORIENTED_EDGE('',*,*,#4536,.F.);
#5756=ORIENTED_EDGE('',*,*,#4537,.T.);
#5757=ORIENTED_EDGE('',*,*,#4538,.F.);
#5758=ORIENTED_EDGE('',*,*,#4534,.F.);
#5759=ORIENTED_EDGE('',*,*,#4539,.F.);
#5760=ORIENTED_EDGE('',*,*,#4540,.T.);
#5761=ORIENTED_EDGE('',*,*,#4541,.F.);
#5762=ORIENTED_EDGE('',*,*,#4537,.F.);
#5763=ORIENTED_EDGE('',*,*,#4542,.F.);
#5764=ORIENTED_EDGE('',*,*,#4543,.T.);
#5765=ORIENTED_EDGE('',*,*,#4544,.F.);
#5766=ORIENTED_EDGE('',*,*,#4540,.F.);
#5767=ORIENTED_EDGE('',*,*,#4545,.F.);
#5768=ORIENTED_EDGE('',*,*,#4546,.F.);
#5769=ORIENTED_EDGE('',*,*,#4547,.F.);
#5770=ORIENTED_EDGE('',*,*,#4543,.F.);
#5771=ORIENTED_EDGE('',*,*,#4548,.F.);
#5772=ORIENTED_EDGE('',*,*,#4549,.T.);
#5773=ORIENTED_EDGE('',*,*,#4550,.F.);
#5774=ORIENTED_EDGE('',*,*,#4549,.F.);
#5775=ORIENTED_EDGE('',*,*,#4462,.T.);
#5776=ORIENTED_EDGE('',*,*,#4551,.T.);
#5777=ORIENTED_EDGE('',*,*,#4552,.T.);
#5778=ORIENTED_EDGE('',*,*,#4553,.F.);
#5779=ORIENTED_EDGE('',*,*,#4439,.T.);
#5780=ORIENTED_EDGE('',*,*,#4554,.F.);
#5781=ORIENTED_EDGE('',*,*,#4555,.F.);
#5782=ORIENTED_EDGE('',*,*,#4556,.T.);
#5783=ORIENTED_EDGE('',*,*,#4490,.T.);
#5784=ORIENTED_EDGE('',*,*,#4557,.T.);
#5785=ORIENTED_EDGE('',*,*,#4555,.T.);
#5786=ORIENTED_EDGE('',*,*,#4558,.F.);
#5787=ORIENTED_EDGE('',*,*,#4467,.T.);
#5788=ORIENTED_EDGE('',*,*,#4559,.F.);
#5789=ORIENTED_EDGE('',*,*,#4560,.F.);
#5790=ORIENTED_EDGE('',*,*,#4561,.T.);
#5791=ORIENTED_EDGE('',*,*,#4518,.T.);
#5792=ORIENTED_EDGE('',*,*,#4562,.T.);
#5793=ORIENTED_EDGE('',*,*,#4560,.T.);
#5794=ORIENTED_EDGE('',*,*,#4563,.F.);
#5795=ORIENTED_EDGE('',*,*,#4495,.T.);
#5796=ORIENTED_EDGE('',*,*,#4564,.F.);
#5797=ORIENTED_EDGE('',*,*,#4565,.F.);
#5798=ORIENTED_EDGE('',*,*,#4566,.T.);
#5799=ORIENTED_EDGE('',*,*,#4546,.T.);
#5800=ORIENTED_EDGE('',*,*,#4567,.T.);
#5801=ORIENTED_EDGE('',*,*,#4565,.T.);
#5802=ORIENTED_EDGE('',*,*,#4568,.F.);
#5803=ORIENTED_EDGE('',*,*,#4523,.T.);
#5804=ORIENTED_EDGE('',*,*,#4569,.F.);
#5805=ORIENTED_EDGE('',*,*,#4552,.F.);
#5806=ORIENTED_EDGE('',*,*,#4570,.T.);
#5807=ORIENTED_EDGE('',*,*,#4438,.T.);
#5808=ORIENTED_EDGE('',*,*,#4442,.T.);
#5809=ORIENTED_EDGE('',*,*,#4445,.T.);
#5810=ORIENTED_EDGE('',*,*,#4448,.T.);
#5811=ORIENTED_EDGE('',*,*,#4451,.T.);
#5812=ORIENTED_EDGE('',*,*,#4454,.T.);
#5813=ORIENTED_EDGE('',*,*,#4457,.T.);
#5814=ORIENTED_EDGE('',*,*,#4460,.T.);
#5815=ORIENTED_EDGE('',*,*,#4463,.T.);
#5816=ORIENTED_EDGE('',*,*,#4553,.T.);
#5817=ORIENTED_EDGE('',*,*,#4569,.T.);
#5818=ORIENTED_EDGE('',*,*,#4522,.T.);
#5819=ORIENTED_EDGE('',*,*,#4526,.T.);
#5820=ORIENTED_EDGE('',*,*,#4529,.T.);
#5821=ORIENTED_EDGE('',*,*,#4532,.T.);
#5822=ORIENTED_EDGE('',*,*,#4535,.T.);
#5823=ORIENTED_EDGE('',*,*,#4538,.T.);
#5824=ORIENTED_EDGE('',*,*,#4541,.T.);
#5825=ORIENTED_EDGE('',*,*,#4544,.T.);
#5826=ORIENTED_EDGE('',*,*,#4547,.T.);
#5827=ORIENTED_EDGE('',*,*,#4568,.T.);
#5828=ORIENTED_EDGE('',*,*,#4564,.T.);
#5829=ORIENTED_EDGE('',*,*,#4494,.T.);
#5830=ORIENTED_EDGE('',*,*,#4498,.T.);
#5831=ORIENTED_EDGE('',*,*,#4501,.T.);
#5832=ORIENTED_EDGE('',*,*,#4504,.T.);
#5833=ORIENTED_EDGE('',*,*,#4507,.T.);
#5834=ORIENTED_EDGE('',*,*,#4510,.T.);
#5835=ORIENTED_EDGE('',*,*,#4513,.T.);
#5836=ORIENTED_EDGE('',*,*,#4516,.T.);
#5837=ORIENTED_EDGE('',*,*,#4519,.T.);
#5838=ORIENTED_EDGE('',*,*,#4563,.T.);
#5839=ORIENTED_EDGE('',*,*,#4559,.T.);
#5840=ORIENTED_EDGE('',*,*,#4466,.T.);
#5841=ORIENTED_EDGE('',*,*,#4470,.T.);
#5842=ORIENTED_EDGE('',*,*,#4473,.T.);
#5843=ORIENTED_EDGE('',*,*,#4476,.T.);
#5844=ORIENTED_EDGE('',*,*,#4479,.T.);
#5845=ORIENTED_EDGE('',*,*,#4482,.T.);
#5846=ORIENTED_EDGE('',*,*,#4485,.T.);
#5847=ORIENTED_EDGE('',*,*,#4488,.T.);
#5848=ORIENTED_EDGE('',*,*,#4491,.T.);
#5849=ORIENTED_EDGE('',*,*,#4558,.T.);
#5850=ORIENTED_EDGE('',*,*,#4554,.T.);
#5851=ORIENTED_EDGE('',*,*,#4550,.T.);
#5852=ORIENTED_EDGE('',*,*,#4436,.T.);
#5853=ORIENTED_EDGE('',*,*,#4556,.F.);
#5854=ORIENTED_EDGE('',*,*,#4557,.F.);
#5855=ORIENTED_EDGE('',*,*,#4489,.T.);
#5856=ORIENTED_EDGE('',*,*,#4486,.T.);
#5857=ORIENTED_EDGE('',*,*,#4483,.T.);
#5858=ORIENTED_EDGE('',*,*,#4480,.T.);
#5859=ORIENTED_EDGE('',*,*,#4477,.T.);
#5860=ORIENTED_EDGE('',*,*,#4474,.T.);
#5861=ORIENTED_EDGE('',*,*,#4471,.T.);
#5862=ORIENTED_EDGE('',*,*,#4468,.T.);
#5863=ORIENTED_EDGE('',*,*,#4464,.T.);
#5864=ORIENTED_EDGE('',*,*,#4561,.F.);
#5865=ORIENTED_EDGE('',*,*,#4562,.F.);
#5866=ORIENTED_EDGE('',*,*,#4517,.T.);
#5867=ORIENTED_EDGE('',*,*,#4514,.T.);
#5868=ORIENTED_EDGE('',*,*,#4511,.T.);
#5869=ORIENTED_EDGE('',*,*,#4508,.T.);
#5870=ORIENTED_EDGE('',*,*,#4505,.T.);
#5871=ORIENTED_EDGE('',*,*,#4502,.T.);
#5872=ORIENTED_EDGE('',*,*,#4499,.T.);
#5873=ORIENTED_EDGE('',*,*,#4496,.T.);
#5874=ORIENTED_EDGE('',*,*,#4492,.T.);
#5875=ORIENTED_EDGE('',*,*,#4566,.F.);
#5876=ORIENTED_EDGE('',*,*,#4567,.F.);
#5877=ORIENTED_EDGE('',*,*,#4545,.T.);
#5878=ORIENTED_EDGE('',*,*,#4542,.T.);
#5879=ORIENTED_EDGE('',*,*,#4539,.T.);
#5880=ORIENTED_EDGE('',*,*,#4536,.T.);
#5881=ORIENTED_EDGE('',*,*,#4533,.T.);
#5882=ORIENTED_EDGE('',*,*,#4530,.T.);
#5883=ORIENTED_EDGE('',*,*,#4527,.T.);
#5884=ORIENTED_EDGE('',*,*,#4524,.T.);
#5885=ORIENTED_EDGE('',*,*,#4520,.T.);
#5886=ORIENTED_EDGE('',*,*,#4570,.F.);
#5887=ORIENTED_EDGE('',*,*,#4551,.F.);
#5888=ORIENTED_EDGE('',*,*,#4461,.T.);
#5889=ORIENTED_EDGE('',*,*,#4458,.T.);
#5890=ORIENTED_EDGE('',*,*,#4455,.T.);
#5891=ORIENTED_EDGE('',*,*,#4452,.T.);
#5892=ORIENTED_EDGE('',*,*,#4449,.T.);
#5893=ORIENTED_EDGE('',*,*,#4446,.T.);
#5894=ORIENTED_EDGE('',*,*,#4443,.T.);
#5895=ORIENTED_EDGE('',*,*,#4440,.T.);
#5896=ORIENTED_EDGE('',*,*,#4548,.T.);
#6921=CYLINDRICAL_SURFACE('',#7982,0.21);
#7098=ADVANCED_FACE('',(#1172),#856,.F.);
#7099=ADVANCED_FACE('',(#1173),#857,.F.);
#7100=ADVANCED_FACE('',(#1174),#858,.F.);
#7101=ADVANCED_FACE('',(#1175),#859,.F.);
#7102=ADVANCED_FACE('',(#1176),#860,.F.);
#7103=ADVANCED_FACE('',(#1177),#861,.F.);
#7104=ADVANCED_FACE('',(#1178),#862,.F.);
#7105=ADVANCED_FACE('',(#1179),#863,.F.);
#7106=ADVANCED_FACE('',(#1180),#864,.F.);
#7107=ADVANCED_FACE('',(#1181),#865,.F.);
#7108=ADVANCED_FACE('',(#1182),#866,.F.);
#7109=ADVANCED_FACE('',(#1183),#867,.F.);
#7110=ADVANCED_FACE('',(#1184),#868,.F.);
#7111=ADVANCED_FACE('',(#1185),#869,.F.);
#7112=ADVANCED_FACE('',(#1186),#870,.F.);
#7113=ADVANCED_FACE('',(#1187),#871,.F.);
#7114=ADVANCED_FACE('',(#1188),#872,.F.);
#7115=ADVANCED_FACE('',(#1189),#873,.F.);
#7116=ADVANCED_FACE('',(#1190),#874,.F.);
#7117=ADVANCED_FACE('',(#1191),#875,.F.);
#7118=ADVANCED_FACE('',(#1192),#876,.F.);
#7119=ADVANCED_FACE('',(#1193),#877,.F.);
#7120=ADVANCED_FACE('',(#1194),#878,.F.);
#7121=ADVANCED_FACE('',(#1195),#879,.F.);
#7122=ADVANCED_FACE('',(#1196),#880,.F.);
#7123=ADVANCED_FACE('',(#1197),#881,.F.);
#7124=ADVANCED_FACE('',(#1198),#882,.F.);
#7125=ADVANCED_FACE('',(#1199),#883,.F.);
#7126=ADVANCED_FACE('',(#1200),#884,.F.);
#7127=ADVANCED_FACE('',(#1201),#885,.F.);
#7128=ADVANCED_FACE('',(#1202),#886,.F.);
#7129=ADVANCED_FACE('',(#1203),#887,.F.);
#7130=ADVANCED_FACE('',(#1204),#888,.F.);
#7131=ADVANCED_FACE('',(#1205),#889,.F.);
#7132=ADVANCED_FACE('',(#1206),#890,.F.);
#7133=ADVANCED_FACE('',(#1207),#891,.F.);
#7134=ADVANCED_FACE('',(#1208),#6921,.F.);
#7135=ADVANCED_FACE('',(#1209),#892,.T.);
#7136=ADVANCED_FACE('',(#1210),#893,.T.);
#7137=ADVANCED_FACE('',(#1211),#894,.T.);
#7138=ADVANCED_FACE('',(#1212),#895,.T.);
#7139=ADVANCED_FACE('',(#1213),#896,.T.);
#7140=ADVANCED_FACE('',(#1214),#897,.T.);
#7141=ADVANCED_FACE('',(#1215),#898,.T.);
#7142=ADVANCED_FACE('',(#1216),#899,.T.);
#7143=ADVANCED_FACE('',(#1217,#690),#900,.T.);
#7144=ADVANCED_FACE('',(#1218,#691),#901,.F.);
#7377=CLOSED_SHELL('',(#7098,#7099,#7100,#7101,#7102,#7103,#7104,#7105,
#7106,#7107,#7108,#7109,#7110,#7111,#7112,#7113,#7114,#7115,#7116,#7117,
#7118,#7119,#7120,#7121,#7122,#7123,#7124,#7125,#7126,#7127,#7128,#7129,
#7130,#7131,#7132,#7133,#7134,#7135,#7136,#7137,#7138,#7139,#7140,#7141,
#7142,#7143,#7144));
#7945=AXIS2_PLACEMENT_3D('',#11284,#9111,#9112);
#7946=AXIS2_PLACEMENT_3D('',#11285,#9113,#9114);
#7947=AXIS2_PLACEMENT_3D('',#11294,#9119,#9120);
#7948=AXIS2_PLACEMENT_3D('',#11300,#9124,#9125);
#7949=AXIS2_PLACEMENT_3D('',#11306,#9129,#9130);
#7950=AXIS2_PLACEMENT_3D('',#11312,#9134,#9135);
#7951=AXIS2_PLACEMENT_3D('',#11318,#9139,#9140);
#7952=AXIS2_PLACEMENT_3D('',#11324,#9144,#9145);
#7953=AXIS2_PLACEMENT_3D('',#11330,#9149,#9150);
#7954=AXIS2_PLACEMENT_3D('',#11336,#9154,#9155);
#7955=AXIS2_PLACEMENT_3D('',#11342,#9159,#9160);
#7956=AXIS2_PLACEMENT_3D('',#11351,#9165,#9166);
#7957=AXIS2_PLACEMENT_3D('',#11357,#9170,#9171);
#7958=AXIS2_PLACEMENT_3D('',#11363,#9175,#9176);
#7959=AXIS2_PLACEMENT_3D('',#11369,#9180,#9181);
#7960=AXIS2_PLACEMENT_3D('',#11375,#9185,#9186);
#7961=AXIS2_PLACEMENT_3D('',#11381,#9190,#9191);
#7962=AXIS2_PLACEMENT_3D('',#11387,#9195,#9196);
#7963=AXIS2_PLACEMENT_3D('',#11393,#9200,#9201);
#7964=AXIS2_PLACEMENT_3D('',#11399,#9205,#9206);
#7965=AXIS2_PLACEMENT_3D('',#11408,#9211,#9212);
#7966=AXIS2_PLACEMENT_3D('',#11414,#9216,#9217);
#7967=AXIS2_PLACEMENT_3D('',#11420,#9221,#9222);
#7968=AXIS2_PLACEMENT_3D('',#11426,#9226,#9227);
#7969=AXIS2_PLACEMENT_3D('',#11432,#9231,#9232);
#7970=AXIS2_PLACEMENT_3D('',#11438,#9236,#9237);
#7971=AXIS2_PLACEMENT_3D('',#11444,#9241,#9242);
#7972=AXIS2_PLACEMENT_3D('',#11450,#9246,#9247);
#7973=AXIS2_PLACEMENT_3D('',#11456,#9251,#9252);
#7974=AXIS2_PLACEMENT_3D('',#11465,#9257,#9258);
#7975=AXIS2_PLACEMENT_3D('',#11471,#9262,#9263);
#7976=AXIS2_PLACEMENT_3D('',#11477,#9267,#9268);
#7977=AXIS2_PLACEMENT_3D('',#11483,#9272,#9273);
#7978=AXIS2_PLACEMENT_3D('',#11489,#9277,#9278);
#7979=AXIS2_PLACEMENT_3D('',#11495,#9282,#9283);
#7980=AXIS2_PLACEMENT_3D('',#11501,#9287,#9288);
#7981=AXIS2_PLACEMENT_3D('',#11507,#9292,#9293);
#7982=AXIS2_PLACEMENT_3D('',#11513,#9297,#9298);
#7983=AXIS2_PLACEMENT_3D('',#11515,#9299,#9300);
#7984=AXIS2_PLACEMENT_3D('',#11518,#9302,#9303);
#7985=AXIS2_PLACEMENT_3D('',#11519,#9304,#9305);
#7986=AXIS2_PLACEMENT_3D('',#11525,#9309,#9310);
#7987=AXIS2_PLACEMENT_3D('',#11531,#9314,#9315);
#7988=AXIS2_PLACEMENT_3D('',#11534,#9318,#9319);
#7989=AXIS2_PLACEMENT_3D('',#11540,#9323,#9324);
#7990=AXIS2_PLACEMENT_3D('',#11543,#9327,#9328);
#7991=AXIS2_PLACEMENT_3D('',#11549,#9332,#9333);
#7992=AXIS2_PLACEMENT_3D('',#11552,#9336,#9337);
#7993=AXIS2_PLACEMENT_3D('',#11555,#9340,#9341);
#7994=AXIS2_PLACEMENT_3D('',#11556,#9342,#9343);
#9111=DIRECTION('axis',(0.,0.,1.));
#9112=DIRECTION('refdir',(1.,0.,0.));
#9113=DIRECTION('center_axis',(0.,0.,-1.));
#9114=DIRECTION('ref_axis',(0.,1.,0.));
#9115=DIRECTION('',(0.,1.,0.));
#9116=DIRECTION('',(1.,0.,0.));
#9117=DIRECTION('',(0.,-1.,0.));
#9118=DIRECTION('',(1.,0.,0.));
#9119=DIRECTION('center_axis',(0.,1.,-8.88178419700125E-16));
#9120=DIRECTION('ref_axis',(0.,8.88178419700125E-16,1.));
#9121=DIRECTION('',(0.,8.88178419700125E-16,1.));
#9122=DIRECTION('',(1.,0.,0.));
#9123=DIRECTION('',(0.,-8.88178419700125E-16,-1.));
#9124=DIRECTION('center_axis',(0.,-7.40148683083439E-16,-1.));
#9125=DIRECTION('ref_axis',(0.,1.,-7.40148683083439E-16));
#9126=DIRECTION('',(0.,1.,-7.40148683083439E-16));
#9127=DIRECTION('',(1.,0.,0.));
#9128=DIRECTION('',(0.,-1.,7.40148683083439E-16));
#9129=DIRECTION('center_axis',(0.,-0.707106781186547,-0.707106781186548));
#9130=DIRECTION('ref_axis',(0.,0.707106781186548,-0.707106781186547));
#9131=DIRECTION('',(0.,0.707106781186548,-0.707106781186547));
#9132=DIRECTION('',(1.,0.,0.));
#9133=DIRECTION('',(0.,-0.707106781186548,0.707106781186547));
#9134=DIRECTION('center_axis',(0.,-1.,2.77555756156289E-16));
#9135=DIRECTION('ref_axis',(0.,-2.77555756156289E-16,-1.));
#9136=DIRECTION('',(0.,-2.77555756156289E-16,-1.));
#9137=DIRECTION('',(1.,0.,0.));
#9138=DIRECTION('',(0.,2.77555756156289E-16,1.));
#9139=DIRECTION('center_axis',(0.,-0.707106781186547,0.707106781186548));
#9140=DIRECTION('ref_axis',(0.,-0.707106781186548,-0.707106781186547));
#9141=DIRECTION('',(0.,-0.707106781186548,-0.707106781186547));
#9142=DIRECTION('',(1.,0.,0.));
#9143=DIRECTION('',(0.,0.707106781186548,0.707106781186547));
#9144=DIRECTION('center_axis',(0.,7.40148683083438E-16,1.));
#9145=DIRECTION('ref_axis',(0.,-1.,7.40148683083438E-16));
#9146=DIRECTION('',(0.,-1.,7.40148683083438E-16));
#9147=DIRECTION('',(1.,0.,0.));
#9148=DIRECTION('',(0.,1.,-7.40148683083438E-16));
#9149=DIRECTION('center_axis',(0.,1.,-4.44089209850063E-16));
#9150=DIRECTION('ref_axis',(0.,4.44089209850063E-16,1.));
#9151=DIRECTION('',(0.,4.44089209850063E-16,1.));
#9152=DIRECTION('',(1.,0.,0.));
#9153=DIRECTION('',(0.,-4.44089209850063E-16,-1.));
#9154=DIRECTION('center_axis',(0.,2.41352831440251E-16,1.));
#9155=DIRECTION('ref_axis',(0.,-1.,2.41352831440251E-16));
#9156=DIRECTION('',(0.,-1.,2.41352831440251E-16));
#9157=DIRECTION('',(-1.,0.,0.));
#9158=DIRECTION('',(0.,1.,-2.41352831440251E-16));
#9159=DIRECTION('center_axis',(0.,-1.,2.41352831440251E-16));
#9160=DIRECTION('ref_axis',(0.,-2.41352831440251E-16,-1.));
#9161=DIRECTION('',(0.,-2.41352831440251E-16,-1.));
#9162=DIRECTION('',(1.,0.,0.));
#9163=DIRECTION('',(0.,2.41352831440251E-16,1.));
#9164=DIRECTION('',(1.,0.,0.));
#9165=DIRECTION('center_axis',(0.,0.,-1.));
#9166=DIRECTION('ref_axis',(0.,1.,0.));
#9167=DIRECTION('',(0.,1.,0.));
#9168=DIRECTION('',(1.,0.,0.));
#9169=DIRECTION('',(0.,-1.,0.));
#9170=DIRECTION('center_axis',(0.,-1.,0.));
#9171=DIRECTION('ref_axis',(0.,0.,-1.));
#9172=DIRECTION('',(0.,0.,-1.));
#9173=DIRECTION('',(1.,0.,0.));
#9174=DIRECTION('',(0.,0.,1.));
#9175=DIRECTION('center_axis',(0.,-0.707106781186547,0.707106781186548));
#9176=DIRECTION('ref_axis',(0.,-0.707106781186548,-0.707106781186547));
#9177=DIRECTION('',(0.,-0.707106781186548,-0.707106781186547));
#9178=DIRECTION('',(1.,0.,0.));
#9179=DIRECTION('',(0.,0.707106781186548,0.707106781186547));
#9180=DIRECTION('center_axis',(0.,0.,1.));
#9181=DIRECTION('ref_axis',(0.,-1.,0.));
#9182=DIRECTION('',(0.,-1.,0.));
#9183=DIRECTION('',(1.,0.,0.));
#9184=DIRECTION('',(0.,1.,0.));
#9185=DIRECTION('center_axis',(0.,0.707106781186548,0.707106781186547));
#9186=DIRECTION('ref_axis',(0.,-0.707106781186547,0.707106781186548));
#9187=DIRECTION('',(0.,-0.707106781186547,0.707106781186548));
#9188=DIRECTION('',(1.,0.,0.));
#9189=DIRECTION('',(0.,0.707106781186547,-0.707106781186548));
#9190=DIRECTION('center_axis',(0.,1.,0.));
#9191=DIRECTION('ref_axis',(0.,0.,1.));
#9192=DIRECTION('',(0.,0.,1.));
#9193=DIRECTION('',(1.,0.,0.));
#9194=DIRECTION('',(0.,0.,-1.));
#9195=DIRECTION('center_axis',(0.,0.,-1.));
#9196=DIRECTION('ref_axis',(0.,1.,0.));
#9197=DIRECTION('',(0.,1.,0.));
#9198=DIRECTION('',(1.,0.,0.));
#9199=DIRECTION('',(0.,-1.,0.));
#9200=DIRECTION('center_axis',(0.,1.,-2.41352831440251E-16));
#9201=DIRECTION('ref_axis',(0.,2.41352831440251E-16,1.));
#9202=DIRECTION('',(0.,2.41352831440251E-16,1.));
#9203=DIRECTION('',(-1.,0.,0.));
#9204=DIRECTION('',(0.,-2.41352831440251E-16,-1.));
#9205=DIRECTION('center_axis',(0.,0.,1.));
#9206=DIRECTION('ref_axis',(0.,-1.,0.));
#9207=DIRECTION('',(0.,-1.,0.));
#9208=DIRECTION('',(1.,0.,0.));
#9209=DIRECTION('',(0.,1.,0.));
#9210=DIRECTION('',(1.,0.,0.));
#9211=DIRECTION('center_axis',(0.,-1.,0.));
#9212=DIRECTION('ref_axis',(0.,0.,-1.));
#9213=DIRECTION('',(0.,0.,-1.));
#9214=DIRECTION('',(1.,0.,0.));
#9215=DIRECTION('',(0.,0.,1.));
#9216=DIRECTION('center_axis',(0.,0.,1.));
#9217=DIRECTION('ref_axis',(0.,-1.,0.));
#9218=DIRECTION('',(0.,-1.,0.));
#9219=DIRECTION('',(1.,0.,0.));
#9220=DIRECTION('',(0.,1.,0.));
#9221=DIRECTION('center_axis',(0.,0.707106781186548,0.707106781186548));
#9222=DIRECTION('ref_axis',(0.,-0.707106781186548,0.707106781186548));
#9223=DIRECTION('',(0.,-0.707106781186548,0.707106781186548));
#9224=DIRECTION('',(1.,0.,0.));
#9225=DIRECTION('',(0.,0.707106781186548,-0.707106781186548));
#9226=DIRECTION('center_axis',(0.,1.,0.));
#9227=DIRECTION('ref_axis',(0.,0.,1.));
#9228=DIRECTION('',(0.,0.,1.));
#9229=DIRECTION('',(1.,0.,0.));
#9230=DIRECTION('',(0.,0.,-1.));
#9231=DIRECTION('center_axis',(0.,0.707106781186548,-0.707106781186547));
#9232=DIRECTION('ref_axis',(0.,0.707106781186547,0.707106781186548));
#9233=DIRECTION('',(0.,0.707106781186547,0.707106781186548));
#9234=DIRECTION('',(1.,0.,0.));
#9235=DIRECTION('',(0.,-0.707106781186547,-0.707106781186548));
#9236=DIRECTION('center_axis',(0.,-7.40148683083438E-16,-1.));
#9237=DIRECTION('ref_axis',(0.,1.,-7.40148683083438E-16));
#9238=DIRECTION('',(0.,1.,-7.40148683083438E-16));
#9239=DIRECTION('',(1.,0.,0.));
#9240=DIRECTION('',(0.,-1.,7.40148683083438E-16));
#9241=DIRECTION('center_axis',(0.,-1.,0.));
#9242=DIRECTION('ref_axis',(0.,0.,-1.));
#9243=DIRECTION('',(0.,0.,-1.));
#9244=DIRECTION('',(1.,0.,0.));
#9245=DIRECTION('',(0.,0.,1.));
#9246=DIRECTION('center_axis',(0.,0.,-1.));
#9247=DIRECTION('ref_axis',(0.,1.,0.));
#9248=DIRECTION('',(0.,1.,0.));
#9249=DIRECTION('',(-1.,0.,0.));
#9250=DIRECTION('',(0.,-1.,0.));
#9251=DIRECTION('center_axis',(0.,1.,0.));
#9252=DIRECTION('ref_axis',(0.,0.,1.));
#9253=DIRECTION('',(0.,0.,1.));
#9254=DIRECTION('',(1.,0.,0.));
#9255=DIRECTION('',(0.,0.,-1.));
#9256=DIRECTION('',(1.,0.,0.));
#9257=DIRECTION('center_axis',(0.,0.,1.));
#9258=DIRECTION('ref_axis',(0.,-1.,0.));
#9259=DIRECTION('',(0.,-1.,0.));
#9260=DIRECTION('',(1.,0.,0.));
#9261=DIRECTION('',(0.,1.,0.));
#9262=DIRECTION('center_axis',(0.,1.,0.));
#9263=DIRECTION('ref_axis',(0.,0.,1.));
#9264=DIRECTION('',(0.,0.,1.));
#9265=DIRECTION('',(1.,0.,0.));
#9266=DIRECTION('',(0.,0.,-1.));
#9267=DIRECTION('center_axis',(0.,0.707106781186547,-0.707106781186548));
#9268=DIRECTION('ref_axis',(0.,0.707106781186548,0.707106781186547));
#9269=DIRECTION('',(0.,0.707106781186548,0.707106781186547));
#9270=DIRECTION('',(1.,0.,0.));
#9271=DIRECTION('',(0.,-0.707106781186548,-0.707106781186547));
#9272=DIRECTION('center_axis',(0.,0.,-1.));
#9273=DIRECTION('ref_axis',(0.,1.,0.));
#9274=DIRECTION('',(0.,1.,0.));
#9275=DIRECTION('',(1.,0.,0.));
#9276=DIRECTION('',(0.,-1.,0.));
#9277=DIRECTION('center_axis',(0.,-0.707106781186547,-0.707106781186548));
#9278=DIRECTION('ref_axis',(0.,0.707106781186548,-0.707106781186547));
#9279=DIRECTION('',(0.,0.707106781186548,-0.707106781186547));
#9280=DIRECTION('',(1.,0.,0.));
#9281=DIRECTION('',(0.,-0.707106781186548,0.707106781186547));
#9282=DIRECTION('center_axis',(0.,-1.,0.));
#9283=DIRECTION('ref_axis',(0.,0.,-1.));
#9284=DIRECTION('',(0.,0.,-1.));
#9285=DIRECTION('',(1.,0.,0.));
#9286=DIRECTION('',(0.,0.,1.));
#9287=DIRECTION('center_axis',(0.,0.,1.));
#9288=DIRECTION('ref_axis',(0.,-1.,0.));
#9289=DIRECTION('',(0.,-1.,0.));
#9290=DIRECTION('',(1.,0.,0.));
#9291=DIRECTION('',(0.,1.,0.));
#9292=DIRECTION('center_axis',(0.,-1.,0.));
#9293=DIRECTION('ref_axis',(0.,0.,-1.));
#9294=DIRECTION('',(0.,0.,-1.));
#9295=DIRECTION('',(-1.,0.,0.));
#9296=DIRECTION('',(0.,0.,1.));
#9297=DIRECTION('center_axis',(1.,0.,0.));
#9298=DIRECTION('ref_axis',(0.,0.,-1.));
#9299=DIRECTION('center_axis',(1.,0.,0.));
#9300=DIRECTION('ref_axis',(0.,0.,-1.));
#9301=DIRECTION('',(1.,0.,0.));
#9302=DIRECTION('center_axis',(-1.,0.,0.));
#9303=DIRECTION('ref_axis',(0.,0.,-1.));
#9304=DIRECTION('center_axis',(0.,1.,0.));
#9305=DIRECTION('ref_axis',(0.,0.,1.));
#9306=DIRECTION('',(0.,0.,1.));
#9307=DIRECTION('',(1.,0.,0.));
#9308=DIRECTION('',(0.,0.,1.));
#9309=DIRECTION('center_axis',(0.,1.,0.));
#9310=DIRECTION('ref_axis',(0.,0.,1.));
#9311=DIRECTION('',(0.,0.,1.));
#9312=DIRECTION('',(1.,0.,0.));
#9313=DIRECTION('',(0.,0.,1.));
#9314=DIRECTION('center_axis',(0.,0.,-1.));
#9315=DIRECTION('ref_axis',(0.,1.,0.));
#9316=DIRECTION('',(0.,1.,0.));
#9317=DIRECTION('',(0.,1.,0.));
#9318=DIRECTION('center_axis',(0.,0.,-1.));
#9319=DIRECTION('ref_axis',(0.,1.,0.));
#9320=DIRECTION('',(0.,1.,0.));
#9321=DIRECTION('',(1.,0.,0.));
#9322=DIRECTION('',(0.,1.,0.));
#9323=DIRECTION('center_axis',(0.,-1.,0.));
#9324=DIRECTION('ref_axis',(0.,0.,-1.));
#9325=DIRECTION('',(0.,0.,-1.));
#9326=DIRECTION('',(0.,0.,-1.));
#9327=DIRECTION('center_axis',(0.,-1.,0.));
#9328=DIRECTION('ref_axis',(0.,0.,-1.));
#9329=DIRECTION('',(0.,0.,-1.));
#9330=DIRECTION('',(1.,0.,0.));
#9331=DIRECTION('',(0.,0.,-1.));
#9332=DIRECTION('center_axis',(0.,0.,1.));
#9333=DIRECTION('ref_axis',(0.,-1.,0.));
#9334=DIRECTION('',(0.,-1.,0.));
#9335=DIRECTION('',(0.,-1.,0.));
#9336=DIRECTION('center_axis',(0.,0.,1.));
#9337=DIRECTION('ref_axis',(0.,-1.,0.));
#9338=DIRECTION('',(0.,-1.,0.));
#9339=DIRECTION('',(0.,-1.,0.));
#9340=DIRECTION('center_axis',(1.,0.,0.));
#9341=DIRECTION('ref_axis',(0.,0.,-1.));
#9342=DIRECTION('center_axis',(1.,0.,0.));
#9343=DIRECTION('ref_axis',(0.,0.,-1.));
#11284=CARTESIAN_POINT('',(0.,0.,0.));
#11285=CARTESIAN_POINT('Origin',(-0.1,0.82,-0.3));
#11286=CARTESIAN_POINT('',(0.,0.82,-0.3));
#11287=CARTESIAN_POINT('',(0.,1.,-0.3));
#11288=CARTESIAN_POINT('',(0.,0.41,-0.3));
#11289=CARTESIAN_POINT('',(40.,0.82,-0.3));
#11290=CARTESIAN_POINT('',(-0.1,0.82,-0.3));
#11291=CARTESIAN_POINT('',(40.,1.,-0.3));
#11292=CARTESIAN_POINT('',(40.,0.41,-0.3));
#11293=CARTESIAN_POINT('',(-0.05,1.,-0.3));
#11294=CARTESIAN_POINT('Origin',(-0.1,0.82,-0.55));
#11295=CARTESIAN_POINT('',(0.,0.82,-0.55));
#11296=CARTESIAN_POINT('',(0.,0.82,-0.275));
#11297=CARTESIAN_POINT('',(40.,0.82,-0.55));
#11298=CARTESIAN_POINT('',(-0.1,0.82,-0.55));
#11299=CARTESIAN_POINT('',(40.,0.82,-0.275));
#11300=CARTESIAN_POINT('Origin',(-0.1,0.67,-0.55));
#11301=CARTESIAN_POINT('',(0.,0.67,-0.55));
#11302=CARTESIAN_POINT('',(0.,0.335,-0.55));
#11303=CARTESIAN_POINT('',(40.,0.67,-0.55));
#11304=CARTESIAN_POINT('',(-0.1,0.67,-0.55));
#11305=CARTESIAN_POINT('',(40.,0.335,-0.55));
#11306=CARTESIAN_POINT('Origin',(-0.1,0.42,-0.3));
#11307=CARTESIAN_POINT('',(0.,0.42,-0.3));
#11308=CARTESIAN_POINT('',(0.,0.24,-0.12));
#11309=CARTESIAN_POINT('',(40.,0.42,-0.3));
#11310=CARTESIAN_POINT('',(-0.1,0.42,-0.3));
#11311=CARTESIAN_POINT('',(40.,0.24,-0.12));
#11312=CARTESIAN_POINT('Origin',(-0.1,0.42,0.3));
#11313=CARTESIAN_POINT('',(0.,0.42,0.3));
#11314=CARTESIAN_POINT('',(0.,0.42,0.15));
#11315=CARTESIAN_POINT('',(40.,0.42,0.3));
#11316=CARTESIAN_POINT('',(-0.1,0.42,0.3));
#11317=CARTESIAN_POINT('',(40.,0.42,0.15));
#11318=CARTESIAN_POINT('Origin',(-0.1,0.67,0.55));
#11319=CARTESIAN_POINT('',(0.,0.67,0.55));
#11320=CARTESIAN_POINT('',(6.93889390390723E-18,0.365,0.245));
#11321=CARTESIAN_POINT('',(40.,0.67,0.55));
#11322=CARTESIAN_POINT('',(-0.1,0.67,0.55));
#11323=CARTESIAN_POINT('',(40.,0.365,0.245));
#11324=CARTESIAN_POINT('Origin',(-0.1,0.82,0.55));
#11325=CARTESIAN_POINT('',(0.,0.82,0.55));
#11326=CARTESIAN_POINT('',(0.,0.41,0.55));
#11327=CARTESIAN_POINT('',(40.,0.82,0.55));
#11328=CARTESIAN_POINT('',(-0.1,0.82,0.55));
#11329=CARTESIAN_POINT('',(40.,0.41,0.55));
#11330=CARTESIAN_POINT('Origin',(-0.1,0.82,0.3));
#11331=CARTESIAN_POINT('',(0.,0.82,0.3));
#11332=CARTESIAN_POINT('',(0.,0.82,0.15));
#11333=CARTESIAN_POINT('',(40.,0.82,0.3));
#11334=CARTESIAN_POINT('',(-0.1,0.82,0.3));
#11335=CARTESIAN_POINT('',(40.,0.82,0.15));
#11336=CARTESIAN_POINT('Origin',(-0.1,1.05,0.3));
#11337=CARTESIAN_POINT('',(0.,1.,0.3));
#11338=CARTESIAN_POINT('',(0.,0.525,0.3));
#11339=CARTESIAN_POINT('',(40.,1.,0.3));
#11340=CARTESIAN_POINT('',(-0.05,1.,0.3));
#11341=CARTESIAN_POINT('',(40.,0.525,0.3));
#11342=CARTESIAN_POINT('Origin',(-0.1,-0.3,-0.82));
#11343=CARTESIAN_POINT('',(0.,-0.3,-0.82));
#11344=CARTESIAN_POINT('',(0.,-0.3,-1.));
#11345=CARTESIAN_POINT('',(0.,-0.3,-0.41));
#11346=CARTESIAN_POINT('',(40.,-0.3,-0.82));
#11347=CARTESIAN_POINT('',(-0.1,-0.3,-0.82));
#11348=CARTESIAN_POINT('',(40.,-0.3,-1.));
#11349=CARTESIAN_POINT('',(40.,-0.3,-0.41));
#11350=CARTESIAN_POINT('',(-0.05,-0.3,-1.));
#11351=CARTESIAN_POINT('Origin',(-0.1,-0.55,-0.82));
#11352=CARTESIAN_POINT('',(0.,-0.55,-0.82));
#11353=CARTESIAN_POINT('',(0.,-0.275,-0.82));
#11354=CARTESIAN_POINT('',(40.,-0.55,-0.82));
#11355=CARTESIAN_POINT('',(-0.1,-0.55,-0.82));
#11356=CARTESIAN_POINT('',(40.,-0.275,-0.82));
#11357=CARTESIAN_POINT('Origin',(-0.1,-0.55,-0.67));
#11358=CARTESIAN_POINT('',(0.,-0.55,-0.67));
#11359=CARTESIAN_POINT('',(0.,-0.55,-0.335));
#11360=CARTESIAN_POINT('',(40.,-0.55,-0.67));
#11361=CARTESIAN_POINT('',(-0.1,-0.55,-0.67));
#11362=CARTESIAN_POINT('',(40.,-0.55,-0.335));
#11363=CARTESIAN_POINT('Origin',(-0.1,-0.3,-0.42));
#11364=CARTESIAN_POINT('',(0.,-0.3,-0.42));
#11365=CARTESIAN_POINT('',(0.,-0.12,-0.24));
#11366=CARTESIAN_POINT('',(40.,-0.3,-0.42));
#11367=CARTESIAN_POINT('',(-0.1,-0.3,-0.42));
#11368=CARTESIAN_POINT('',(40.,-0.12,-0.24));
#11369=CARTESIAN_POINT('Origin',(-0.1,0.3,-0.42));
#11370=CARTESIAN_POINT('',(0.,0.3,-0.42));
#11371=CARTESIAN_POINT('',(0.,0.15,-0.42));
#11372=CARTESIAN_POINT('',(40.,0.3,-0.42));
#11373=CARTESIAN_POINT('',(-0.1,0.3,-0.42));
#11374=CARTESIAN_POINT('',(40.,0.15,-0.42));
#11375=CARTESIAN_POINT('Origin',(-0.1,0.55,-0.67));
#11376=CARTESIAN_POINT('',(0.,0.55,-0.67));
#11377=CARTESIAN_POINT('',(0.,0.245,-0.365));
#11378=CARTESIAN_POINT('',(40.,0.55,-0.67));
#11379=CARTESIAN_POINT('',(-0.1,0.55,-0.67));
#11380=CARTESIAN_POINT('',(40.,0.245,-0.365));
#11381=CARTESIAN_POINT('Origin',(-0.1,0.55,-0.82));
#11382=CARTESIAN_POINT('',(0.,0.55,-0.82));
#11383=CARTESIAN_POINT('',(0.,0.55,-0.41));
#11384=CARTESIAN_POINT('',(40.,0.55,-0.82));
#11385=CARTESIAN_POINT('',(-0.1,0.55,-0.82));
#11386=CARTESIAN_POINT('',(40.,0.55,-0.41));
#11387=CARTESIAN_POINT('Origin',(-0.1,0.3,-0.82));
#11388=CARTESIAN_POINT('',(0.,0.3,-0.82));
#11389=CARTESIAN_POINT('',(0.,0.15,-0.82));
#11390=CARTESIAN_POINT('',(40.,0.3,-0.82));
#11391=CARTESIAN_POINT('',(-0.1,0.3,-0.82));
#11392=CARTESIAN_POINT('',(40.,0.15,-0.82));
#11393=CARTESIAN_POINT('Origin',(-0.1,0.3,-1.05));
#11394=CARTESIAN_POINT('',(0.,0.3,-1.));
#11395=CARTESIAN_POINT('',(0.,0.3,-0.525));
#11396=CARTESIAN_POINT('',(40.,0.3,-1.));
#11397=CARTESIAN_POINT('',(-0.05,0.3,-1.));
#11398=CARTESIAN_POINT('',(40.,0.3,-0.525));
#11399=CARTESIAN_POINT('Origin',(-0.1,-0.82,0.3));
#11400=CARTESIAN_POINT('',(0.,-0.82,0.3));
#11401=CARTESIAN_POINT('',(0.,-1.,0.3));
#11402=CARTESIAN_POINT('',(0.,-0.41,0.3));
#11403=CARTESIAN_POINT('',(40.,-0.82,0.3));
#11404=CARTESIAN_POINT('',(-0.1,-0.82,0.3));
#11405=CARTESIAN_POINT('',(40.,-1.,0.3));
#11406=CARTESIAN_POINT('',(40.,-0.41,0.3));
#11407=CARTESIAN_POINT('',(-0.05,-1.,0.3));
#11408=CARTESIAN_POINT('Origin',(-0.1,-0.82,0.55));
#11409=CARTESIAN_POINT('',(0.,-0.82,0.55));
#11410=CARTESIAN_POINT('',(0.,-0.82,0.275));
#11411=CARTESIAN_POINT('',(40.,-0.82,0.55));
#11412=CARTESIAN_POINT('',(-0.1,-0.82,0.55));
#11413=CARTESIAN_POINT('',(40.,-0.82,0.275));
#11414=CARTESIAN_POINT('Origin',(-0.1,-0.67,0.55));
#11415=CARTESIAN_POINT('',(0.,-0.67,0.55));
#11416=CARTESIAN_POINT('',(0.,-0.335,0.55));
#11417=CARTESIAN_POINT('',(40.,-0.67,0.55));
#11418=CARTESIAN_POINT('',(-0.1,-0.67,0.55));
#11419=CARTESIAN_POINT('',(40.,-0.335,0.55));
#11420=CARTESIAN_POINT('Origin',(-0.1,-0.42,0.3));
#11421=CARTESIAN_POINT('',(0.,-0.42,0.3));
#11422=CARTESIAN_POINT('',(-6.93889390390723E-18,-0.24,0.12));
#11423=CARTESIAN_POINT('',(40.,-0.42,0.3));
#11424=CARTESIAN_POINT('',(-0.1,-0.42,0.3));
#11425=CARTESIAN_POINT('',(40.,-0.24,0.12));
#11426=CARTESIAN_POINT('Origin',(-0.1,-0.42,-0.3));
#11427=CARTESIAN_POINT('',(0.,-0.42,-0.3));
#11428=CARTESIAN_POINT('',(0.,-0.42,-0.15));
#11429=CARTESIAN_POINT('',(40.,-0.42,-0.3));
#11430=CARTESIAN_POINT('',(-0.1,-0.42,-0.3));
#11431=CARTESIAN_POINT('',(40.,-0.42,-0.15));
#11432=CARTESIAN_POINT('Origin',(-0.1,-0.67,-0.55));
#11433=CARTESIAN_POINT('',(0.,-0.67,-0.55));
#11434=CARTESIAN_POINT('',(0.,-0.365,-0.245));
#11435=CARTESIAN_POINT('',(40.,-0.67,-0.55));
#11436=CARTESIAN_POINT('',(-0.1,-0.67,-0.55));
#11437=CARTESIAN_POINT('',(40.,-0.365,-0.245));
#11438=CARTESIAN_POINT('Origin',(-0.1,-0.82,-0.55));
#11439=CARTESIAN_POINT('',(0.,-0.82,-0.55));
#11440=CARTESIAN_POINT('',(0.,-0.41,-0.55));
#11441=CARTESIAN_POINT('',(40.,-0.82,-0.55));
#11442=CARTESIAN_POINT('',(-0.1,-0.82,-0.55));
#11443=CARTESIAN_POINT('',(40.,-0.41,-0.55));
#11444=CARTESIAN_POINT('Origin',(-0.1,-0.82,-0.3));
#11445=CARTESIAN_POINT('',(0.,-0.82,-0.3));
#11446=CARTESIAN_POINT('',(0.,-0.82,-0.15));
#11447=CARTESIAN_POINT('',(40.,-0.82,-0.3));
#11448=CARTESIAN_POINT('',(-0.1,-0.82,-0.3));
#11449=CARTESIAN_POINT('',(40.,-0.82,-0.15));
#11450=CARTESIAN_POINT('Origin',(-0.1,-1.05,-0.3));
#11451=CARTESIAN_POINT('',(0.,-1.,-0.3));
#11452=CARTESIAN_POINT('',(0.,-0.525,-0.3));
#11453=CARTESIAN_POINT('',(40.,-1.,-0.3));
#11454=CARTESIAN_POINT('',(-0.05,-1.,-0.3));
#11455=CARTESIAN_POINT('',(40.,-0.525,-0.3));
#11456=CARTESIAN_POINT('Origin',(-0.1,0.3,0.82));
#11457=CARTESIAN_POINT('',(0.,0.3,0.82));
#11458=CARTESIAN_POINT('',(0.,0.3,1.));
#11459=CARTESIAN_POINT('',(0.,0.3,0.41));
#11460=CARTESIAN_POINT('',(40.,0.3,0.82));
#11461=CARTESIAN_POINT('',(-0.1,0.3,0.82));
#11462=CARTESIAN_POINT('',(40.,0.3,1.));
#11463=CARTESIAN_POINT('',(40.,0.3,0.41));
#11464=CARTESIAN_POINT('',(-0.05,0.3,1.));
#11465=CARTESIAN_POINT('Origin',(-0.1,0.55,0.82));
#11466=CARTESIAN_POINT('',(0.,0.55,0.82));
#11467=CARTESIAN_POINT('',(0.,0.275,0.82));
#11468=CARTESIAN_POINT('',(40.,0.55,0.82));
#11469=CARTESIAN_POINT('',(-0.1,0.55,0.82));
#11470=CARTESIAN_POINT('',(40.,0.275,0.82));
#11471=CARTESIAN_POINT('Origin',(-0.1,0.55,0.67));
#11472=CARTESIAN_POINT('',(0.,0.55,0.67));
#11473=CARTESIAN_POINT('',(0.,0.55,0.335));
#11474=CARTESIAN_POINT('',(40.,0.55,0.67));
#11475=CARTESIAN_POINT('',(-0.1,0.55,0.67));
#11476=CARTESIAN_POINT('',(40.,0.55,0.335));
#11477=CARTESIAN_POINT('Origin',(-0.1,0.3,0.42));
#11478=CARTESIAN_POINT('',(0.,0.3,0.42));
#11479=CARTESIAN_POINT('',(6.93889390390723E-18,0.12,0.24));
#11480=CARTESIAN_POINT('',(40.,0.3,0.42));
#11481=CARTESIAN_POINT('',(-0.1,0.3,0.42));
#11482=CARTESIAN_POINT('',(40.,0.12,0.24));
#11483=CARTESIAN_POINT('Origin',(-0.1,-0.3,0.42));
#11484=CARTESIAN_POINT('',(0.,-0.3,0.42));
#11485=CARTESIAN_POINT('',(0.,-0.15,0.42));
#11486=CARTESIAN_POINT('',(40.,-0.3,0.42));
#11487=CARTESIAN_POINT('',(-0.1,-0.3,0.42));
#11488=CARTESIAN_POINT('',(40.,-0.15,0.42));
#11489=CARTESIAN_POINT('Origin',(-0.1,-0.55,0.67));
#11490=CARTESIAN_POINT('',(0.,-0.55,0.67));
#11491=CARTESIAN_POINT('',(6.93889390390723E-18,-0.245,0.365));
#11492=CARTESIAN_POINT('',(40.,-0.55,0.67));
#11493=CARTESIAN_POINT('',(-0.1,-0.55,0.67));
#11494=CARTESIAN_POINT('',(40.,-0.245,0.365));
#11495=CARTESIAN_POINT('Origin',(-0.1,-0.55,0.82));
#11496=CARTESIAN_POINT('',(0.,-0.55,0.82));
#11497=CARTESIAN_POINT('',(0.,-0.55,0.41));
#11498=CARTESIAN_POINT('',(40.,-0.55,0.82));
#11499=CARTESIAN_POINT('',(-0.1,-0.55,0.82));
#11500=CARTESIAN_POINT('',(40.,-0.55,0.41));
#11501=CARTESIAN_POINT('Origin',(-0.1,-0.3,0.82));
#11502=CARTESIAN_POINT('',(0.,-0.3,0.82));
#11503=CARTESIAN_POINT('',(0.,-0.15,0.82));
#11504=CARTESIAN_POINT('',(40.,-0.3,0.82));
#11505=CARTESIAN_POINT('',(-0.1,-0.3,0.82));
#11506=CARTESIAN_POINT('',(40.,-0.15,0.82));
#11507=CARTESIAN_POINT('Origin',(-0.1,-0.3,1.05));
#11508=CARTESIAN_POINT('',(0.,-0.3,1.));
#11509=CARTESIAN_POINT('',(0.,-0.3,0.525));
#11510=CARTESIAN_POINT('',(40.,-0.3,1.));
#11511=CARTESIAN_POINT('',(-0.05,-0.3,1.));
#11512=CARTESIAN_POINT('',(40.,-0.3,0.525));
#11513=CARTESIAN_POINT('Origin',(-0.1,0.,0.));
#11514=CARTESIAN_POINT('',(0.,-2.57175827820944E-17,0.21));
#11515=CARTESIAN_POINT('Origin',(0.,0.,0.));
#11516=CARTESIAN_POINT('',(40.,2.57175827820944E-17,0.21));
#11517=CARTESIAN_POINT('',(-0.1,-2.57175827820944E-17,0.21));
#11518=CARTESIAN_POINT('Origin',(40.,0.,0.));
#11519=CARTESIAN_POINT('Origin',(0.,1.,-1.));
#11520=CARTESIAN_POINT('',(0.,1.,1.));
#11521=CARTESIAN_POINT('',(0.,1.,-1.));
#11522=CARTESIAN_POINT('',(40.,1.,1.));
#11523=CARTESIAN_POINT('',(0.,1.,1.));
#11524=CARTESIAN_POINT('',(40.,1.,-1.));
#11525=CARTESIAN_POINT('Origin',(0.,1.,-1.));
#11526=CARTESIAN_POINT('',(40.,1.,-1.));
#11527=CARTESIAN_POINT('',(40.,1.,-1.));
#11528=CARTESIAN_POINT('',(0.,1.,-1.));
#11529=CARTESIAN_POINT('',(0.,1.,-1.));
#11530=CARTESIAN_POINT('',(0.,1.,-1.));
#11531=CARTESIAN_POINT('Origin',(0.,-1.,-1.));
#11532=CARTESIAN_POINT('',(0.,-1.,-1.));
#11533=CARTESIAN_POINT('',(40.,-1.,-1.));
#11534=CARTESIAN_POINT('Origin',(0.,-1.,-1.));
#11535=CARTESIAN_POINT('',(40.,-1.,-1.));
#11536=CARTESIAN_POINT('',(40.,-1.,-1.));
#11537=CARTESIAN_POINT('',(0.,-1.,-1.));
#11538=CARTESIAN_POINT('',(0.,-1.,-1.));
#11539=CARTESIAN_POINT('',(0.,-1.,-1.));
#11540=CARTESIAN_POINT('Origin',(0.,-1.,1.));
#11541=CARTESIAN_POINT('',(0.,-1.,1.));
#11542=CARTESIAN_POINT('',(40.,-1.,1.));
#11543=CARTESIAN_POINT('Origin',(0.,-1.,1.));
#11544=CARTESIAN_POINT('',(40.,-1.,1.));
#11545=CARTESIAN_POINT('',(40.,-1.,1.));
#11546=CARTESIAN_POINT('',(0.,-1.,1.));
#11547=CARTESIAN_POINT('',(0.,-1.,1.));
#11548=CARTESIAN_POINT('',(0.,-1.,1.));
#11549=CARTESIAN_POINT('Origin',(0.,1.,1.));
#11550=CARTESIAN_POINT('',(0.,1.,1.));
#11551=CARTESIAN_POINT('',(40.,1.,1.));
#11552=CARTESIAN_POINT('Origin',(0.,1.,1.));
#11553=CARTESIAN_POINT('',(40.,1.,1.));
#11554=CARTESIAN_POINT('',(0.,1.,1.));
#11555=CARTESIAN_POINT('Origin',(40.,0.,0.));
#11556=CARTESIAN_POINT('Origin',(0.,0.,0.));
#12749=UNCERTAINTY_MEASURE_WITH_UNIT(LENGTH_MEASURE(0.001),#12805,
'DISTANCE_ACCURACY_VALUE',
'Maximum model space distance between geometric entities at asserted c
onnectivities');
#12768=UNCERTAINTY_MEASURE_WITH_UNIT(LENGTH_MEASURE(0.001),#12805,
'DISTANCE_ACCURACY_VALUE',
'Maximum model space distance between geometric entities at asserted c
onnectivities');
#12785=(
GEOMETRIC_REPRESENTATION_CONTEXT(3)
GLOBAL_UNCERTAINTY_ASSIGNED_CONTEXT((#12749))
GLOBAL_UNIT_ASSIGNED_CONTEXT((#12805,#12807,#12808))
REPRESENTATION_CONTEXT('','3D')
);
#12804=(
GEOMETRIC_REPRESENTATION_CONTEXT(3)
GLOBAL_UNCERTAINTY_ASSIGNED_CONTEXT((#12768))
GLOBAL_UNIT_ASSIGNED_CONTEXT((#12805,#12807,#12808))
REPRESENTATION_CONTEXT('','3D')
);
#12805=(
LENGTH_UNIT()
NAMED_UNIT(*)
SI_UNIT(.CENTI.,.METRE.)
);
#12807=(
NAMED_UNIT(*)
PLANE_ANGLE_UNIT()
SI_UNIT($,.RADIAN.)
);
#12808=(
NAMED_UNIT(*)
SI_UNIT($,.STERADIAN.)
SOLID_ANGLE_UNIT()
);
#12825=SHAPE_DEFINITION_REPRESENTATION(#12860,#13015);
#12860=PRODUCT_DEFINITION_SHAPE('',$,#13051);
#13015=SHAPE_REPRESENTATION('',(#7945),#12785);
#13034=PRODUCT_DEFINITION_CONTEXT('part definition',#13141,'design');
#13051=PRODUCT_DEFINITION('Slotted Extrusion - 20 x 20 x 400 mm',
'Slotted Extrusion - 20 x 20 x 400 mm',#13086,#13034);
#13086=PRODUCT_DEFINITION_FORMATION('',$,#13159);
#13141=APPLICATION_CONTEXT(
'Core Data for Automotive Mechanical Design Process');
#13142=PRODUCT_CONTEXT('part definition',#13141,'mechanical');
#13159=PRODUCT('Slotted Extrusion - 20 x 20 x 400 mm',
'Slotted Extrusion - 20 x 20 x 400 mm',
'Slotted Extrusion - 20 x 20 x 400 mm',(#13142));
#13227=COLOUR_RGB('Light Blue',0.38,0.62,0.78);
#13228=FILL_AREA_STYLE_COLOUR('',#13227);
#13229=FILL_AREA_STYLE('',(#13228));
#13230=SURFACE_STYLE_FILL_AREA(#13229);
#13231=SURFACE_SIDE_STYLE('',(#13230));
#13232=SURFACE_STYLE_USAGE(.BOTH.,#13231);
#13233=PRESENTATION_STYLE_ASSIGNMENT((#13232));
ENDSEC;
END-ISO-10303-21;
